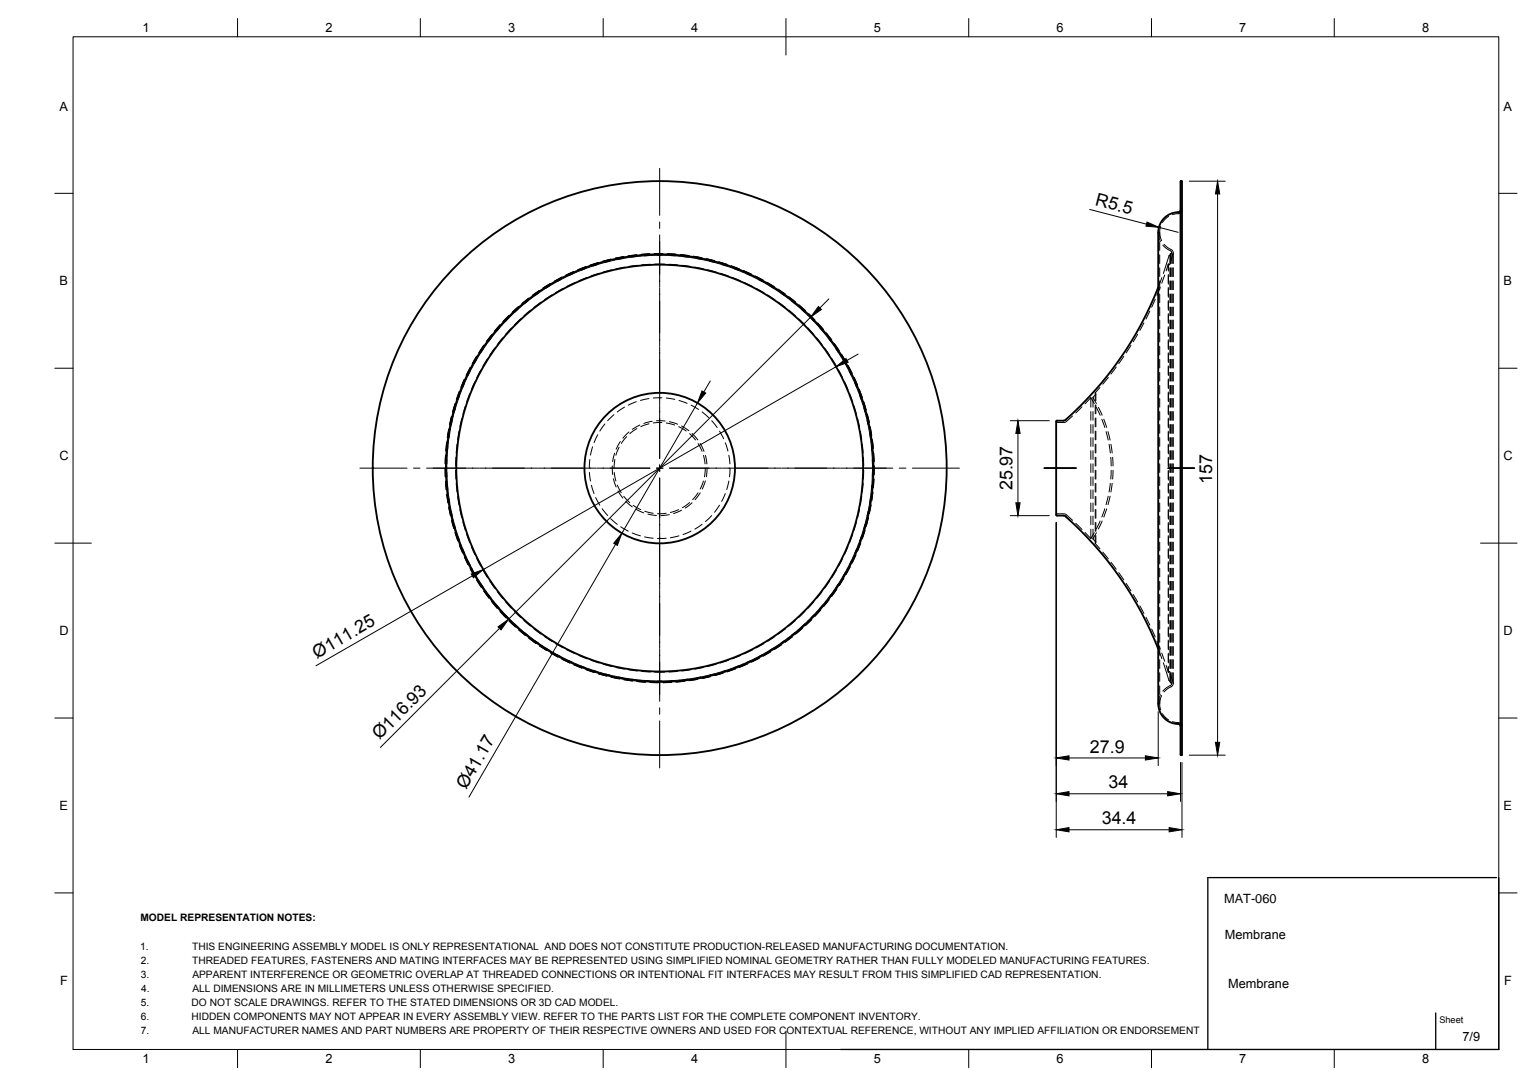
ISO-10303-21;
HEADER;
FILE_DESCRIPTION (('STEP AP214'),
    '1' );
FILE_NAME ('Membrane.step',
    '2026-10-29T23:46:56',
    ( '' ),
    ( '' ),
    'SwSTEP 2.0',
    'SolidWorks 2020',
    '' );
FILE_SCHEMA (( 'AUTOMOTIVE_DESIGN' ));
ENDSEC;

DATA;
#42=FILL_AREA_STYLE ('',( #30241 ) ) ;
#55=ORIENTED_EDGE ( 'NONE', *, *, #8639, .T. ) ;
#70=CIRCLE ( 'NONE', #12126, 59.80962967564905597 ) ;
#78=CARTESIAN_POINT ( 'NONE',  ( 21.09785597605719332, 15.24673779880127356, 47.04930799450051637 ) ) ;
#85=DIRECTION ( 'NONE',  ( 0.000000000000000000, 1.000000000000000000, -0.000000000000000000 ) ) ;
#87=AXIS2_PLACEMENT_3D ( 'NONE', #1243, #25723, #26032 ) ;
#88=DIRECTION ( 'NONE',  ( 0.000000000000000000, 1.000000000000000000, -0.000000000000000000 ) ) ;
#94=DIRECTION ( 'NONE',  ( 0.000000000000000000, 0.000000000000000000, 1.000000000000000000 ) ) ;
#128=DIRECTION ( 'NONE',  ( 0.000000000000000000, 0.000000000000000000, -1.000000000000000000 ) ) ;
#170=DIRECTION ( 'NONE',  ( -1.096245967261381435E-16, 0.000000000000000000, 1.000000000000000000 ) ) ;
#202=ORIENTED_EDGE ( 'NONE', *, *, #17749, .F. ) ;
#214=ORIENTED_EDGE ( 'NONE', *, *, #14166, .F. ) ;
#226=EDGE_CURVE ( 'NONE', #1958, #14944, #28442, .T. ) ;
#255=ORIENTED_EDGE ( 'NONE', *, *, #25304, .F. ) ;
#258=AXIS2_PLACEMENT_3D ( 'NONE', #29211, #16405, #11331 ) ;
#260=AXIS2_PLACEMENT_3D ( 'NONE', #19965, #12767, #2897 ) ;
#268=CARTESIAN_POINT ( 'NONE',  ( 21.09785597605719332, 14.58544108513610027, 34.31529089466609150 ) ) ;
#269=DIRECTION ( 'NONE',  ( -1.000000000000000000, 0.000000000000000000, 0.000000000000000000 ) ) ;
#307=CARTESIAN_POINT ( 'NONE',  ( 21.09785597605720042, -16.63545420775220407, -31.35069200549948221 ) ) ;
#329=EDGE_CURVE ( 'NONE', #6215, #18606, #11548, .T. ) ;
#347=DIRECTION ( 'NONE',  ( 0.000000000000000000, 0.000000000000000000, 1.000000000000000000 ) ) ;
#389=FACE_OUTER_BOUND ( 'NONE', #5612, .T. ) ;
#394=AXIS2_PLACEMENT_3D ( 'NONE', #24259, #4561, #23933 ) ;
#415=EDGE_LOOP ( 'NONE', ( #28557, #12550, #27414, #27034 ) ) ;
#427=DIRECTION ( 'NONE',  ( 0.000000000000000000, 0.000000000000000000, 1.000000000000000000 ) ) ;
#506=CARTESIAN_POINT ( 'NONE',  ( 21.09785597605719332, 14.77310068074637961, 33.81390520620020368 ) ) ;
#529=VERTEX_POINT ( 'NONE', #29166 ) ;
#549=ADVANCED_FACE ( 'NONE', ( #24556 ), #24396, .T. ) ;
#571=CARTESIAN_POINT ( 'NONE',  ( 21.09785597605719332, 7.237299147902269247, 47.04930799450051637 ) ) ;
#608=DIRECTION ( 'NONE',  ( 0.000000000000000000, 0.000000000000000000, -1.000000000000000000 ) ) ;
#653=CARTESIAN_POINT ( 'NONE',  ( 21.09785597605719332, 6.717634499306958773, 26.77287239547234066 ) ) ;
#660=AXIS2_PLACEMENT_3D ( 'NONE', #13969, #11830, #16569 ) ;
#664=CIRCLE ( 'NONE', #5918, 5.499019513592785735 ) ;
#673=CARTESIAN_POINT ( 'NONE',  ( -3.635677172050030048, -13.30632128221581212, 97.21573990761679340 ) ) ;
#675=DIRECTION ( 'NONE',  ( 0.000000000000000000, 0.000000000000000000, -1.000000000000000000 ) ) ;
#712=CIRCLE ( 'NONE', #19588, 0.6000000000000033085 ) ;
#722=CARTESIAN_POINT ( 'NONE',  ( 21.09785597605719332, 7.237299147902269247, 27.58963108451947832 ) ) ;
#726=DIRECTION ( 'NONE',  ( 0.000000000000000000, 0.000000000000000000, -1.000000000000000000 ) ) ;
#730=AXIS2_PLACEMENT_3D ( 'NONE', #24703, #6978, #12237 ) ;
#756=VERTEX_POINT ( 'NONE', #30915 ) ;
#769=CARTESIAN_POINT ( 'NONE',  ( 21.09785597605719332, 17.36451738380053555, 59.83349819502753775 ) ) ;
#806=DIRECTION ( 'NONE',  ( 0.000000000000000000, 0.000000000000000000, 1.000000000000000000 ) ) ;
#824=( GEOMETRIC_REPRESENTATION_CONTEXT ( 3 ) GLOBAL_UNCERTAINTY_ASSIGNED_CONTEXT ( ( #14065 ) ) GLOBAL_UNIT_ASSIGNED_CONTEXT ( ( #9888, #7594, #28105 ) ) REPRESENTATION_CONTEXT ( 'NONE', 'WORKASPACE' ) );
#834=DIRECTION ( 'NONE',  ( 0.000000000000000000, 0.000000000000000000, -1.000000000000000000 ) ) ;
#838=DIRECTION ( 'NONE',  ( 0.000000000000000000, 0.000000000000000000, -1.000000000000000000 ) ) ;
#846=CARTESIAN_POINT ( 'NONE',  ( 75.12562691325334185, -13.30632128221581212, 61.52060788219942822 ) ) ;
#851=CARTESIAN_POINT ( 'NONE',  ( 21.09785597605720042, -14.04221034894631615, -11.81388374861560386 ) ) ;
#989=CARTESIAN_POINT ( 'NONE',  ( -29.06857593705904108, -13.30632128221581212, 71.78284114260779347 ) ) ;
#994=CARTESIAN_POINT ( 'NONE',  ( 21.09785597605719332, 17.16451738380053271, 59.83349819502753775 ) ) ;
#1017=AXIS2_PLACEMENT_3D ( 'NONE', #653, #5424, #10682 ) ;
#1046=CARTESIAN_POINT ( 'NONE',  ( 21.09785597605720042, -16.73545420775220194, 47.04930799450051637 ) ) ;
#1047=DIRECTION ( 'NONE',  ( 0.000000000000000000, 0.000000000000000000, -1.000000000000000000 ) ) ;
#1059=DIRECTION ( 'NONE',  ( -0.000000000000000000, -1.000000000000000000, -0.000000000000000000 ) ) ;
#1070=EDGE_CURVE ( 'NONE', #20704, #4372, #13505, .T. ) ;
#1093=ORIENTED_EDGE ( 'NONE', *, *, #29693, .T. ) ;
#1113=DIRECTION ( 'NONE',  ( -0.000000000000000000, -1.000000000000000000, -0.000000000000000000 ) ) ;
#1117=EDGE_LOOP ( 'NONE', ( #3032, #2932, #25525, #9085 ) ) ;
#1139=AXIS2_PLACEMENT_3D ( 'NONE', #16369, #23761, #6373 ) ;
#1145=CARTESIAN_POINT ( 'NONE',  ( -27.33830150920369206, -13.30632128221581389, 19.07865907559173380 ) ) ;
#1157=VERTEX_POINT ( 'NONE', #4269 ) ;
#1163=EDGE_LOOP ( 'NONE', ( #13477, #4955, #25769, #255 ) ) ;
#1166=EDGE_CURVE ( 'NONE', #14445, #6352, #14609, .T. ) ;
#1168=FACE_OUTER_BOUND ( 'NONE', #32182, .T. ) ;
#1172=CARTESIAN_POINT ( 'NONE',  ( 21.09785597605720042, -14.54791319078308653, -11.41466734444011877 ) ) ;
#1181=AXIS2_PLACEMENT_3D ( 'NONE', #4062, #6693, #31807 ) ;
#1211=DIRECTION ( 'NONE',  ( 1.000000000000000000, 0.000000000000000000, 0.000000000000000000 ) ) ;
#1219=CARTESIAN_POINT ( 'NONE',  ( 21.09785597605719332, 17.16451738380053271, 47.04930799450051637 ) ) ;
#1243=CARTESIAN_POINT ( 'NONE',  ( 21.09785597605720753, -16.03545420775219910, 111.5493079945005235 ) ) ;
#1271=AXIS2_PLACEMENT_3D ( 'NONE', #17739, #12013, #20208 ) ;
#1318=ORIENTED_EDGE ( 'NONE', *, *, #9258, .F. ) ;
#1322=DIRECTION ( 'NONE',  ( -0.000000000000000000, -1.000000000000000000, -0.000000000000000000 ) ) ;
#1327=CARTESIAN_POINT ( 'NONE',  ( 39.85850837550805892, -13.74047052604243113, -8.200871005067009278 ) ) ;
#1354=DIRECTION ( 'NONE',  ( 0.000000000000000000, 0.000000000000000000, 1.000000000000000000 ) ) ;
#1374=DIRECTION ( 'NONE',  ( 0.000000000000000000, 0.000000000000000000, -1.000000000000000000 ) ) ;
#1376=ADVANCED_FACE ( 'NONE', ( #20171 ), #28437, .T. ) ;
#1399=EDGE_CURVE ( 'NONE', #18054, #15162, #3087, .T. ) ;
#1427=CARTESIAN_POINT ( 'NONE',  ( 21.09785597605720042, -13.37218737171702543, 47.04930799450051637 ) ) ;
#1455=DIRECTION ( 'NONE',  ( 0.000000000000000000, 1.000000000000000000, -0.000000000000000000 ) ) ;
#1456=CIRCLE ( 'NONE', #7745, 59.44168675549763492 ) ;
#1481=CARTESIAN_POINT ( 'NONE',  ( 76.91070899933976079, -13.30632128221581212, 43.39636530629569933 ) ) ;
#1486=CARTESIAN_POINT ( 'NONE',  ( 24.90860134598588616, -13.74047052604243468, -11.17459240441505841 ) ) ;
#1496=TOROIDAL_SURFACE ( 'NONE', #19845, 78.39999999999999147, 0.1000000000000014350 ) ;
#1506=AXIS2_PLACEMENT_3D ( 'NONE', #10006, #14769, #22786 ) ;
#1511=CARTESIAN_POINT ( 'NONE',  ( 21.09785597605720042, -17.03545420775220265, 47.04930799450051637 ) ) ;
#1520=DIRECTION ( 'NONE',  ( 3.629881133194233264E-17, 0.9550631830613039996, -0.2964022880492153122 ) ) ;
#1528=ORIENTED_EDGE ( 'NONE', *, *, #15802, .T. ) ;
#1531=DIRECTION ( 'NONE',  ( 1.000000000000000000, 0.000000000000000000, -1.224646799147353207E-16 ) ) ;
#1533=CARTESIAN_POINT ( 'NONE',  ( 21.09785597605720042, -13.68834655544033652, 47.04930799450051637 ) ) ;
#1540=AXIS2_PLACEMENT_3D ( 'NONE', #4446, #23662, #19040 ) ;
#1547=DIRECTION ( 'NONE',  ( 1.000000000000000000, 0.000000000000000000, -1.224646799147353207E-16 ) ) ;
#1549=CARTESIAN_POINT ( 'NONE',  ( 21.09785597605720753, -17.03545420775220265, 117.6483275080933169 ) ) ;
#1590=DIRECTION ( 'NONE',  ( -0.000000000000000000, -1.000000000000000000, -0.000000000000000000 ) ) ;
#1624=CIRCLE ( 'NONE', #32023, 69.59901951359279337 ) ;
#1655=CARTESIAN_POINT ( 'NONE',  ( 64.96297466771234497, -13.74047052604243646, 85.52521890125203186 ) ) ;
#1658=CARTESIAN_POINT ( 'NONE',  ( 21.09785597605720042, -13.64309448858209528, 47.04930799450051637 ) ) ;
#1672=FACE_OUTER_BOUND ( 'NONE', #25999, .T. ) ;
#1674=AXIS2_PLACEMENT_3D ( 'NONE', #9447, #19766, #14863 ) ;
#1683=ORIENTED_EDGE ( 'NONE', *, *, #28988, .F. ) ;
#1723=ORIENTED_EDGE ( 'NONE', *, *, #1399, .F. ) ;
#1735=AXIS2_PLACEMENT_3D ( 'NONE', #18661, #1113, #9306 ) ;
#1760=ORIENTED_EDGE ( 'NONE', *, *, #5361, .T. ) ;
#1806=ADVANCED_FACE ( 'NONE', ( #16019 ), #14235, .F. ) ;
#1807=CIRCLE ( 'NONE', #31687, 1.000000000000000888 ) ;
#1817=DIRECTION ( 'NONE',  ( 0.000000000000000000, 0.000000000000000000, -1.000000000000000000 ) ) ;
#1820=FACE_OUTER_BOUND ( 'NONE', #8386, .T. ) ;
#1832=FACE_OUTER_BOUND ( 'NONE', #19834, .T. ) ;
#1842=CARTESIAN_POINT ( 'NONE',  ( 21.09785597605719332, -13.74048473023143835, -11.17459240385188934 ) ) ;
#1846=ORIENTED_EDGE ( 'NONE', *, *, #12585, .F. ) ;
#1852=DIRECTION ( 'NONE',  ( 0.000000000000000000, 0.000000000000000000, -1.000000000000000000 ) ) ;
#1866=ORIENTED_EDGE ( 'NONE', *, *, #20239, .T. ) ;
#1904=AXIS2_PLACEMENT_3D ( 'NONE', #31595, #14029, #11568 ) ;
#1916=CARTESIAN_POINT ( 'NONE',  ( 1.883339950622007652, 7.264443105416139801, 47.04930799450051637 ) ) ;
#1942=CARTESIAN_POINT ( 'NONE',  ( 21.09785597605720042, -13.98292989133646103, 47.04930799450051637 ) ) ;
#1958=VERTEX_POINT ( 'NONE', #4188 ) ;
#1965=DIRECTION ( 'NONE',  ( 0.000000000000000000, 0.000000000000000000, -1.000000000000000000 ) ) ;
#1977=CARTESIAN_POINT ( 'NONE',  ( 39.85850837550807313, -13.74047052604243824, 102.2994869940680616 ) ) ;
#2054=DIRECTION ( 'NONE',  ( -0.000000000000000000, 0.000000000000000000, 1.000000000000000000 ) ) ;
#2060=DIRECTION ( 'NONE',  ( 0.000000000000000000, 1.000000000000000000, -0.000000000000000000 ) ) ;
#2074=AXIS2_PLACEMENT_3D ( 'NONE', #27150, #7137, #7301 ) ;
#2140=ORIENTED_EDGE ( 'NONE', *, *, #22896, .T. ) ;
#2158=AXIS2_PLACEMENT_3D ( 'NONE', #22995, #5122, #12845 ) ;
#2167=DIRECTION ( 'NONE',  ( 0.000000000000000000, 0.000000000000000000, 1.000000000000000000 ) ) ;
#2172=CARTESIAN_POINT ( 'NONE',  ( 21.09785597605719332, 6.547041198165487685, 47.04930799450051637 ) ) ;
#2203=DIRECTION ( 'NONE',  ( 1.169615070119505487E-16, -0.2964022880492245271, 0.9550631830613013351 ) ) ;
#2204=TOROIDAL_SURFACE ( 'NONE', #22655, 64.50000000000000000, 5.099019513592785380 ) ;
#2222=DIRECTION ( 'NONE',  ( 1.000000000000000000, 0.000000000000000000, -1.224646799147353207E-16 ) ) ;
#2226=DIRECTION ( 'NONE',  ( 0.000000000000000000, 0.000000000000000000, -1.000000000000000000 ) ) ;
#2233=PRODUCT_DEFINITION_SHAPE ( 'NONE', 'NONE',  #31780 ) ;
#2234=ORIENTED_EDGE ( 'NONE', *, *, #4882, .T. ) ;
#2241=ORIENTED_EDGE ( 'NONE', *, *, #24153, .T. ) ;
#2247=CIRCLE ( 'NONE', #18498, 55.68770647617149194 ) ;
#2292=ORIENTED_EDGE ( 'NONE', *, *, #24852, .F. ) ;
#2318=CARTESIAN_POINT ( 'NONE',  ( 21.09785597605719332, 17.36451738380053555, 47.04930799450051637 ) ) ;
#2320=CONICAL_SURFACE ( 'NONE', #20662, 58.70143199044622406, 1.269872874662816509 ) ;
#2330=CARTESIAN_POINT ( 'NONE',  ( 21.09785597605720042, -13.59284023713420630, 47.04930799450051637 ) ) ;
#2398=ORIENTED_EDGE ( 'NONE', *, *, #27659, .T. ) ;
#2399=CIRCLE ( 'NONE', #23356, 55.96105416618080142 ) ;
#2404=EDGE_CURVE ( 'NONE', #11885, #27524, #27429, .T. ) ;
#2428=DIRECTION ( 'NONE',  ( -1.000000000000000000, 0.000000000000000000, 0.000000000000000000 ) ) ;
#2447=CARTESIAN_POINT ( 'NONE',  ( 21.09785597605718976, 6.547041198165487685, 67.43013672359793986 ) ) ;
#2453=DIRECTION ( 'NONE',  ( -0.000000000000000000, -1.000000000000000000, -0.000000000000000000 ) ) ;
#2474=ORIENTED_EDGE ( 'NONE', *, *, #3629, .F. ) ;
#2484=EDGE_CURVE ( 'NONE', #20946, #18375, #23232, .T. ) ;
#2515=CIRCLE ( 'NONE', #13073, 58.84990142703892246 ) ;
#2542=CIRCLE ( 'NONE', #20877, 55.68770647617149194 ) ;
#2588=DIRECTION ( 'NONE',  ( 0.000000000000000000, 0.000000000000000000, -1.000000000000000000 ) ) ;
#2595=TOROIDAL_SURFACE ( 'NONE', #29318, 58.88977237527051756, 0.5999999999999987566 ) ;
#2596=ORIENTED_EDGE ( 'NONE', *, *, #6937, .F. ) ;
#2602=CIRCLE ( 'NONE', #5211, 19.45967690998103805 ) ;
#2607=ORIENTED_EDGE ( 'NONE', *, *, #8665, .T. ) ;
#2610=CARTESIAN_POINT ( 'NONE',  ( 21.09785597605720042, -13.87844638871996850, 47.04930799450051637 ) ) ;
#2628=CIRCLE ( 'NONE', #4190, 78.50000000000000000 ) ;
#2646=ORIENTED_EDGE ( 'NONE', *, *, #3109, .T. ) ;
#2653=CARTESIAN_POINT ( 'NONE',  ( 21.09785597605720753, -13.40182760052194588, 102.8325207889781439 ) ) ;
#2683=EDGE_CURVE ( 'NONE', #5958, #20704, #12223, .T. ) ;
#2745=DIRECTION ( 'NONE',  ( -0.000000000000000000, -1.000000000000000000, -0.000000000000000000 ) ) ;
#2768=VECTOR ( 'NONE', #3452, 1000.000000000000114 ) ;
#2774=DIRECTION ( 'NONE',  ( -1.169615070119510171E-16, -0.2964022880492104273, -0.9550631830613055540 ) ) ;
#2816=AXIS2_PLACEMENT_3D ( 'NONE', #19771, #27826, #2226 ) ;
#2853=AXIS2_PLACEMENT_3D ( 'NONE', #13835, #23830, #29087 ) ;
#2857=DIRECTION ( 'NONE',  ( 0.000000000000000000, -1.000000000000000000, 0.000000000000000000 ) ) ;
#2881=AXIS2_PLACEMENT_3D ( 'NONE', #2172, #32370, #4960 ) ;
#2884=AXIS2_PLACEMENT_3D ( 'NONE', #22880, #3008, #5170 ) ;
#2897=DIRECTION ( 'NONE',  ( 0.000000000000000000, 0.000000000000000000, -1.000000000000000000 ) ) ;
#2909=CIRCLE ( 'NONE', #25448, 94.44530576803552435 ) ;
#2918=VECTOR ( 'NONE', #6397, 1000.000000000000000 ) ;
#2932=ORIENTED_EDGE ( 'NONE', *, *, #9760, .T. ) ;
#2936=DIRECTION ( 'NONE',  ( 0.000000000000000000, 0.000000000000000000, -1.000000000000000000 ) ) ;
#2974=ORIENTED_EDGE ( 'NONE', *, *, #30326, .F. ) ;
#3008=DIRECTION ( 'NONE',  ( 0.000000000000000000, 1.000000000000000000, -0.000000000000000000 ) ) ;
#3009=ORIENTED_EDGE ( 'NONE', *, *, #27393, .F. ) ;
#3028=ORIENTED_EDGE ( 'NONE', *, *, #4339, .F. ) ;
#3029=CARTESIAN_POINT ( 'NONE',  ( 21.09785597605719687, -13.30631372918550959, -8.763520691563154941 ) ) ;
#3032=ORIENTED_EDGE ( 'NONE', *, *, #1070, .F. ) ;
#3042=AXIS2_PLACEMENT_3D ( 'NONE', #2653, #7742, #10050 ) ;
#3065=CIRCLE ( 'NONE', #25607, 78.39999999999999147 ) ;
#3067=CIRCLE ( 'NONE', #10926, 19.25826962553310295 ) ;
#3074=ORIENTED_EDGE ( 'NONE', *, *, #2484, .T. ) ;
#3075=DIRECTION ( 'NONE',  ( 0.000000000000000000, 1.000000000000000000, -0.000000000000000000 ) ) ;
#3077=AXIS2_PLACEMENT_3D ( 'NONE', #1533, #1059, #1374 ) ;
#3087=LINE ( 'NONE', #13127, #6941 ) ;
#3109=EDGE_CURVE ( 'NONE', #529, #11769, #28510, .T. ) ;
#3118=CARTESIAN_POINT ( 'NONE',  ( 21.09785597605720042, -13.59284023713420630, 47.04930799450051637 ) ) ;
#3147=TOROIDAL_SURFACE ( 'NONE', #7361, 19.31976987914897848, 0.2000000000000029809 ) ;
#3152=AXIS2_PLACEMENT_3D ( 'NONE', #1511, #6768, #28768 ) ;
#3196=CIRCLE ( 'NONE', #18902, 20.38082872909741994 ) ;
#3197=EDGE_LOOP ( 'NONE', ( #1318, #3565, #29612, #29507 ) ) ;
#3233=DIRECTION ( 'NONE',  ( 0.000000000000000000, 0.000000000000000000, -1.000000000000000000 ) ) ;
#3245=ORIENTED_EDGE ( 'NONE', *, *, #3999, .T. ) ;
#3288=CARTESIAN_POINT ( 'NONE',  ( -34.35522249183560461, -13.30632128221581389, 39.74351294429737891 ) ) ;
#3290=CARTESIAN_POINT ( 'NONE',  ( 99.49785597605720966, -17.03545420775220265, 47.04930799450051637 ) ) ;
#3293=CARTESIAN_POINT ( 'NONE',  ( 21.09785597605720042, -13.37218737171702543, 47.04930799450051637 ) ) ;
#3360=ORIENTED_EDGE ( 'NONE', *, *, #4615, .F. ) ;
#3365=FACE_OUTER_BOUND ( 'NONE', #21547, .T. ) ;
#3366=AXIS2_PLACEMENT_3D ( 'NONE', #9560, #6010, #28811 ) ;
#3385=CARTESIAN_POINT ( 'NONE',  ( 21.09785597605720042, -16.73545420775220194, 47.04930799450051637 ) ) ;
#3408=B_SPLINE_CURVE_WITH_KNOTS ( 'NONE', 3,
 ( #3626, #21171, #31209, #8717, #28427, #30573, #20864, #8087, #5941, #5779, #18397, #25790, #13338, #23335, #846, #10870, #4440, #1481, #21982, #3953, #14296, #16574, #26760, #11834, #9366, #16418, #13974, #14461, #23965, #9038, #4280, #31850, #11497, #26279 ),
 .UNSPECIFIED., .F., .F.,
 ( 4, 2, 2, 2, 2, 2, 2, 2, 2, 2, 2, 2, 2, 2, 2, 2, 4 ),
 ( 0.5000000000000000000, 0.5312500000000000000, 0.5625000000000000000, 0.5937500000000000000, 0.6250000000000000000, 0.6562500000000000000, 0.6875000000000001110, 0.7187500000000002220, 0.7500000000000002220, 0.7812500000000002220, 0.8125000000000002220, 0.8437500000000002220, 0.8750000000000002220, 0.9062500000000002220, 0.9375000000000001110, 0.9687500000000000000, 1.000000000000000000 ),
 .UNSPECIFIED. ) ;
#3414=CIRCLE ( 'NONE', #18103, 58.46397533894063514 ) ;
#3420=CIRCLE ( 'NONE', #23346, 20.58349629884742882 ) ;
#3421=ORIENTED_EDGE ( 'NONE', *, *, #5597, .T. ) ;
#3450=CARTESIAN_POINT ( 'NONE',  ( -15.78477032795855273, -13.30632128221581034, 5.000640598253890623 ) ) ;
#3452=DIRECTION ( 'NONE',  ( 0.000000000000000000, 0.9550631830612811290, 0.2964022880492887535 ) ) ;
#3453=ORIENTED_EDGE ( 'NONE', *, *, #12042, .F. ) ;
#3454=DIRECTION ( 'NONE',  ( 0.000000000000000000, 0.000000000000000000, 1.000000000000000000 ) ) ;
#3455=ORIENTED_EDGE ( 'NONE', *, *, #20389, .T. ) ;
#3457=FACE_OUTER_BOUND ( 'NONE', #20170, .T. ) ;
#3501=ORIENTED_EDGE ( 'NONE', *, *, #25610, .F. ) ;
#3531=DIRECTION ( 'NONE',  ( 0.000000000000000000, 1.000000000000000000, -0.000000000000000000 ) ) ;
#3536=FACE_OUTER_BOUND ( 'NONE', #12646, .T. ) ;
#3540=ORIENTED_EDGE ( 'NONE', *, *, #15853, .F. ) ;
#3544=CARTESIAN_POINT ( 'NONE',  ( 21.09785597605717555, 77.37241625295546044, 131.0041668858331150 ) ) ;
#3565=ORIENTED_EDGE ( 'NONE', *, *, #9477, .F. ) ;
#3573=EDGE_LOOP ( 'NONE', ( #10658, #5418, #25603, #19859 ) ) ;
#3602=AXIS2_PLACEMENT_3D ( 'NONE', #4162, #14189, #1211 ) ;
#3603=CIRCLE ( 'NONE', #20350, 58.09216821878681003 ) ;
#3611=CARTESIAN_POINT ( 'NONE',  ( -12.94741462430177315, -13.30632128221581389, 2.672082950226038367 ) ) ;
#3626=CARTESIAN_POINT ( 'NONE',  ( 21.09785597605719687, -13.30631372918550959, 102.8621366805641770 ) ) ;
#3629=EDGE_CURVE ( 'NONE', #27949, #20704, #24670, .T. ) ;
#3645=LINE ( 'NONE', #25811, #24845 ) ;
#3675=CIRCLE ( 'NONE', #3152, 70.59901951359279337 ) ;
#3686=AXIS2_PLACEMENT_3D ( 'NONE', #10722, #30256, #30584 ) ;
#3703=DIRECTION ( 'NONE',  ( 0.000000000000000000, 0.000000000000000000, -1.000000000000000000 ) ) ;
#3735=DIRECTION ( 'NONE',  ( 0.000000000000000000, 0.000000000000000000, -1.000000000000000000 ) ) ;
#3760=AXIS2_PLACEMENT_3D ( 'NONE', #7446, #17441, #24497 ) ;
#3772=CARTESIAN_POINT ( 'NONE',  ( -12.94741462430176249, -13.30632128221581212, 91.42653303877501969 ) ) ;
#3773=CIRCLE ( 'NONE', #3760, 78.39999999999999147 ) ;
#3784=ORIENTED_EDGE ( 'NONE', *, *, #31237, .F. ) ;
#3785=ORIENTED_EDGE ( 'NONE', *, *, #9760, .F. ) ;
#3792=CARTESIAN_POINT ( 'NONE',  ( 28.71925248772579664, -13.74047052604243291, -10.79927602576051093 ) ) ;
#3800=ADVANCED_FACE ( 'NONE', ( #1820 ), #8372, .F. ) ;
#3802=CARTESIAN_POINT ( 'NONE',  ( 21.09785597605719332, 38.31023907818019580, 47.04930799450051637 ) ) ;
#3813=CARTESIAN_POINT ( 'NONE',  ( 21.09785597605721108, -16.73545420775220194, 125.5493079945005093 ) ) ;
#3822=EDGE_CURVE ( 'NONE', #18054, #23177, #20677, .T. ) ;
#3843=CIRCLE ( 'NONE', #1735, 55.62393233686778160 ) ;
#3864=VERTEX_POINT ( 'NONE', #22325 ) ;
#3915=CIRCLE ( 'NONE', #26990, 78.50000000000000000 ) ;
#3918=AXIS2_PLACEMENT_3D ( 'NONE', #26048, #3075, #30672 ) ;
#3942=ORIENTED_EDGE ( 'NONE', *, *, #14008, .F. ) ;
#3943=CARTESIAN_POINT ( 'NONE',  ( -34.71499704722533153, -13.30632128221581034, 50.70225068270534052 ) ) ;
#3953=CARTESIAN_POINT ( 'NONE',  ( 75.12562691325332764, -13.30632128221581212, 32.57800810680159032 ) ) ;
#3959=CARTESIAN_POINT ( 'NONE',  ( 67.39212317433589305, -13.74047052604243824, 11.53332310724655230 ) ) ;
#3974=ORIENTED_EDGE ( 'NONE', *, *, #10954, .T. ) ;
#3989=DIRECTION ( 'NONE',  ( 0.000000000000000000, 0.000000000000000000, -1.000000000000000000 ) ) ;
#3999=EDGE_CURVE ( 'NONE', #9462, #25082, #8400, .T. ) ;
#4050=DIRECTION ( 'NONE',  ( 0.000000000000000000, 1.000000000000000000, -0.000000000000000000 ) ) ;
#4054=EDGE_LOOP ( 'NONE', ( #31986, #7662, #22931, #16979 ) ) ;
#4062=CARTESIAN_POINT ( 'NONE',  ( 99.49785597605720966, -16.63545420775220052, 47.04930799450051637 ) ) ;
#4113=CARTESIAN_POINT ( 'NONE',  ( 59.57376688280871946, -13.74047052604243646, 3.184189302845370495 ) ) ;
#4116=DIRECTION ( 'NONE',  ( 0.000000000000000000, 1.000000000000000000, -0.000000000000000000 ) ) ;
#4121=CARTESIAN_POINT ( 'NONE',  ( 21.09785597605720753, -13.59284023713420630, 102.7732403313682994 ) ) ;
#4135=AXIS2_PLACEMENT_3D ( 'NONE', #7384, #2453, #12470 ) ;
#4141=DIRECTION ( 'NONE',  ( 0.000000000000000000, 0.000000000000000000, -1.000000000000000000 ) ) ;
#4162=CARTESIAN_POINT ( 'NONE',  ( 21.09785597605719332, 38.31023907818019580, 47.04930799450051637 ) ) ;
#4188=CARTESIAN_POINT ( 'NONE',  ( 21.09785597605721108, -16.63545420775220407, 125.4493079945005150 ) ) ;
#4190=AXIS2_PLACEMENT_3D ( 'NONE', #30921, #5814, #25981 ) ;
#4223=AXIS2_PLACEMENT_3D ( 'NONE', #9362, #19356, #15573 ) ;
#4259=CARTESIAN_POINT ( 'NONE',  ( 21.09785597605719332, 34.11266481626051217, 47.04930799450051637 ) ) ;
#4264=ADVANCED_FACE ( 'NONE', ( #30492 ), #22563, .F. ) ;
#4269=CARTESIAN_POINT ( 'NONE',  ( 21.09785597605719332, 6.671061906060458568, 26.46581169565308755 ) ) ;
#4278=ORIENTED_EDGE ( 'NONE', *, *, #10988, .F. ) ;
#4280=CARTESIAN_POINT ( 'NONE',  ( 35.56915586375611582, -13.30632128221581212, -6.978462942695603743 ) ) ;
#4302=DIRECTION ( 'NONE',  ( 0.000000000000000000, 0.000000000000000000, -1.000000000000000000 ) ) ;
#4303=CARTESIAN_POINT ( 'NONE',  ( 21.09785597605720042, -13.37218737171702543, 47.04930799450051637 ) ) ;
#4331=ORIENTED_EDGE ( 'NONE', *, *, #31682, .T. ) ;
#4339=EDGE_CURVE ( 'NONE', #29876, #31613, #29914, .T. ) ;
#4351=CARTESIAN_POINT ( 'NONE',  ( 21.09785597605720042, -16.03545420775219910, 47.04930799450051637 ) ) ;
#4372=VERTEX_POINT ( 'NONE', #769 ) ;
#4389=DIRECTION ( 'NONE',  ( 0.000000000000000000, 0.000000000000000000, 1.000000000000000000 ) ) ;
#4407=CIRCLE ( 'NONE', #18609, 78.39999999999999147 ) ;
#4431=CARTESIAN_POINT ( 'NONE',  ( 21.09785597605719332, -13.49020584019834601, 105.1414762132873193 ) ) ;
#4435=FACE_OUTER_BOUND ( 'NONE', #24062, .T. ) ;
#4440=CARTESIAN_POINT ( 'NONE',  ( 76.91070899933976079, -13.30632128221581212, 50.70225068270534763 ) ) ;
#4446=CARTESIAN_POINT ( 'NONE',  ( 21.09785597605720042, -13.37218737171702543, 47.04930799450051637 ) ) ;
#4467=CARTESIAN_POINT ( 'NONE',  ( 21.09785597605719332, 17.16451738380053271, 47.04930799450051637 ) ) ;
#4485=CARTESIAN_POINT ( 'NONE',  ( 21.09785597605719332, 14.58544108513610027, 59.78332509433494124 ) ) ;
#4534=AXIS2_PLACEMENT_3D ( 'NONE', #19092, #14200, #29129 ) ;
#4545=EDGE_CURVE ( 'NONE', #14867, #11885, #26250, .T. ) ;
#4560=DIRECTION ( 'NONE',  ( 0.000000000000000000, 0.000000000000000000, -1.000000000000000000 ) ) ;
#4561=DIRECTION ( 'NONE',  ( 0.000000000000000000, -1.000000000000000000, 0.000000000000000000 ) ) ;
#4570=ORIENTED_EDGE ( 'NONE', *, *, #2683, .T. ) ;
#4582=EDGE_LOOP ( 'NONE', ( #10714, #25149, #27986, #22308 ) ) ;
#4607=ADVANCED_FACE ( 'NONE', ( #32423 ), #32015, .F. ) ;
#4615=EDGE_CURVE ( 'NONE', #28177, #11145, #22044, .T. ) ;
#4645=CARTESIAN_POINT ( 'NONE',  ( 21.09785597605719332, 17.16451738380053271, 34.26511779397349500 ) ) ;
#4652=DIRECTION ( 'NONE',  ( 0.000000000000000000, 0.000000000000000000, -1.000000000000000000 ) ) ;
#4657=ORIENTED_EDGE ( 'NONE', *, *, #31935, .F. ) ;
#4668=ORIENTED_EDGE ( 'NONE', *, *, #7760, .T. ) ;
#4681=DIRECTION ( 'NONE',  ( 0.000000000000000000, 0.000000000000000000, -1.000000000000000000 ) ) ;
#4683=FACE_OUTER_BOUND ( 'NONE', #31207, .T. ) ;
#4690=CIRCLE ( 'NONE', #10465, 0.1999999999999987899 ) ;
#4698=CONICAL_SURFACE ( 'NONE', #16239, 20.38082872909741994, 1.021642509542357802 ) ;
#4712=ORIENTED_EDGE ( 'NONE', *, *, #3629, .T. ) ;
#4727=DIRECTION ( 'NONE',  ( 0.000000000000000000, 1.000000000000000000, -0.000000000000000000 ) ) ;
#4760=TOROIDAL_SURFACE ( 'NONE', #10014, 58.86319174311611846, 0.1999999999999984290 ) ;
#4781=DIRECTION ( 'NONE',  ( -1.000000000000000000, 0.000000000000000000, 0.000000000000000000 ) ) ;
#4797=CARTESIAN_POINT ( 'NONE',  ( -25.19641122222149576, -13.74047052604243646, 82.56529288175448755 ) ) ;
#4852=CARTESIAN_POINT ( 'NONE',  ( 21.09785597605719332, 6.717634499306958773, 47.04930799450051637 ) ) ;
#4857=ADVANCED_FACE ( 'NONE', ( #16457 ), #19772, .T. ) ;
#4858=CARTESIAN_POINT ( 'NONE',  ( 21.09785597605720042, -16.03545420775219910, -17.45069200549948718 ) ) ;
#4865=EDGE_LOOP ( 'NONE', ( #26649, #31897, #11347, #7235 ) ) ;
#4873=CIRCLE ( 'NONE', #31611, 0.1000000000000011297 ) ;
#4875=CARTESIAN_POINT ( 'NONE',  ( 21.09785597605719332, 38.31023907818019580, 47.04930799450051637 ) ) ;
#4882=EDGE_CURVE ( 'NONE', #31146, #14944, #16628, .T. ) ;
#4899=DIRECTION ( 'NONE',  ( -0.000000000000000000, -1.000000000000000000, -0.000000000000000000 ) ) ;
#4905=EDGE_CURVE ( 'NONE', #20809, #32483, #26149, .T. ) ;
#4906=CIRCLE ( 'NONE', #32155, 20.38082872909741994 ) ;
#4911=EDGE_LOOP ( 'NONE', ( #8926, #30976, #16052, #8516 ) ) ;
#4940=DIRECTION ( 'NONE',  ( 0.000000000000000000, 0.000000000000000000, -1.000000000000000000 ) ) ;
#4955=ORIENTED_EDGE ( 'NONE', *, *, #15318, .T. ) ;
#4960=DIRECTION ( 'NONE',  ( 0.000000000000000000, 0.000000000000000000, -1.000000000000000000 ) ) ;
#4975=AXIS2_PLACEMENT_3D ( 'NONE', #27104, #17418, #14969 ) ;
#4984=AXIS2_PLACEMENT_3D ( 'NONE', #3293, #15775, #347 ) ;
#4988=AXIS2_PLACEMENT_3D ( 'NONE', #11967, #13956, #23947 ) ;
#4999=CIRCLE ( 'NONE', #25373, 20.58349629884742882 ) ;
#5020=CARTESIAN_POINT ( 'NONE',  ( 21.09785597605720042, -13.68834655544033652, 47.04930799450051637 ) ) ;
#5031=COLOUR_RGB ( '',0.7921568627450980005, 0.8196078431372548767, 0.9333333333333333481 ) ;
#5037=EDGE_CURVE ( 'NONE', #29666, #18375, #30289, .T. ) ;
#5062=CYLINDRICAL_SURFACE ( 'NONE', #6403, 78.50000000000000000 ) ;
#5085=DIRECTION ( 'NONE',  ( 0.000000000000000000, 1.000000000000000000, -0.000000000000000000 ) ) ;
#5094=CARTESIAN_POINT ( 'NONE',  ( 21.09785597605720042, -14.24176827912842391, 47.04930799450051637 ) ) ;
#5103=ORIENTED_EDGE ( 'NONE', *, *, #2404, .T. ) ;
#5107=CIRCLE ( 'NONE', #15592, 0.1999999999999987899 ) ;
#5118=AXIS2_PLACEMENT_3D ( 'NONE', #5677, #23715, #18461 ) ;
#5122=DIRECTION ( 'NONE',  ( 0.000000000000000000, 1.000000000000000000, -0.000000000000000000 ) ) ;
#5137=DIRECTION ( 'NONE',  ( 0.000000000000000000, 0.000000000000000000, -1.000000000000000000 ) ) ;
#5144=CARTESIAN_POINT ( 'NONE',  ( 21.09785597605720042, -16.03545420775220265, -22.54971151909227700 ) ) ;
#5170=DIRECTION ( 'NONE',  ( 0.000000000000000000, 0.000000000000000000, -1.000000000000000000 ) ) ;
#5211=AXIS2_PLACEMENT_3D ( 'NONE', #571, #13061, #10763 ) ;
#5212=DIRECTION ( 'NONE',  ( -0.000000000000000000, -1.000000000000000000, -0.000000000000000000 ) ) ;
#5222=DIRECTION ( 'NONE',  ( 0.000000000000000000, 0.000000000000000000, -1.000000000000000000 ) ) ;
#5248=EDGE_LOOP ( 'NONE', ( #4570, #8141, #13699, #32453 ) ) ;
#5278=CARTESIAN_POINT ( 'NONE',  ( 21.09785597605718976, 7.264443105416139801, 66.26382401993569715 ) ) ;
#5292=FACE_OUTER_BOUND ( 'NONE', #4582, .T. ) ;
#5297=ORIENTED_EDGE ( 'NONE', *, *, #22376, .F. ) ;
#5322=CONICAL_SURFACE ( 'NONE', #12136, 58.70143199044622406, 1.269872874662816509 ) ;
#5335=DIRECTION ( 'NONE',  ( 0.000000000000000000, 0.000000000000000000, -1.000000000000000000 ) ) ;
#5361=EDGE_CURVE ( 'NONE', #29666, #27949, #9849, .T. ) ;
#5376=DIRECTION ( 'NONE',  ( -0.000000000000000000, -1.000000000000000000, -0.000000000000000000 ) ) ;
#5395=ORIENTED_EDGE ( 'NONE', *, *, #21571, .F. ) ;
#5409=ORIENTED_EDGE ( 'NONE', *, *, #30326, .T. ) ;
#5418=ORIENTED_EDGE ( 'NONE', *, *, #22376, .T. ) ;
#5424=DIRECTION ( 'NONE',  ( 1.000000000000000000, 0.000000000000000000, 0.000000000000000000 ) ) ;
#5449=DIRECTION ( 'NONE',  ( 0.000000000000000000, 0.000000000000000000, -1.000000000000000000 ) ) ;
#5463=EDGE_CURVE ( 'NONE', #17607, #29601, #8013, .T. ) ;
#5477=ORIENTED_EDGE ( 'NONE', *, *, #22080, .F. ) ;
#5485=DIRECTION ( 'NONE',  ( 0.000000000000000000, 0.000000000000000000, -1.000000000000000000 ) ) ;
#5486=CIRCLE ( 'NONE', #4975, 1.000000000001013856 ) ;
#5491=ORIENTED_EDGE ( 'NONE', *, *, #26667, .T. ) ;
#5520=DIRECTION ( 'NONE',  ( 3.629881133195132442E-17, 0.9550631830612811290, -0.2964022880492887535 ) ) ;
#5521=ORIENTED_EDGE ( 'NONE', *, *, #329, .T. ) ;
#5560=ADVANCED_FACE ( 'NONE', ( #22769 ), #27175, .T. ) ;
#5577=EDGE_CURVE ( 'NONE', #11769, #22362, #3067, .T. ) ;
#5597=EDGE_CURVE ( 'NONE', #29666, #5958, #15880, .T. ) ;
#5612=EDGE_LOOP ( 'NONE', ( #12655, #6042 ) ) ;
#5649=AXIS2_PLACEMENT_3D ( 'NONE', #8838, #8361, #18358 ) ;
#5677=CARTESIAN_POINT ( 'NONE',  ( 21.09785597605719332, 38.31023907818019580, 47.04930799450051637 ) ) ;
#5691=CARTESIAN_POINT ( 'NONE',  ( 21.09785597605720042, -16.03545420775220265, 47.04930799450051637 ) ) ;
#5701=CARTESIAN_POINT ( 'NONE',  ( 21.09785597605719332, 7.881678200673685630, 47.04930799450051637 ) ) ;
#5757=ORIENTED_EDGE ( 'NONE', *, *, #12585, .T. ) ;
#5771=CARTESIAN_POINT ( 'NONE',  ( 21.09785597605719332, -13.49020584019834601, -11.04286022428629188 ) ) ;
#5779=CARTESIAN_POINT ( 'NONE',  ( 63.14652337230385371, -13.30632128221581389, 83.93193429851626775 ) ) ;
#5814=DIRECTION ( 'NONE',  ( -0.000000000000000000, -1.000000000000000000, -0.000000000000000000 ) ) ;
#5832=DIRECTION ( 'NONE',  ( -1.000000000000000000, 0.000000000000000000, -1.224646799147353207E-16 ) ) ;
#5834=ADVANCED_FACE ( 'NONE', ( #32271 ), #19941, .F. ) ;
#5835=CARTESIAN_POINT ( 'NONE',  ( 21.09785597605720042, -13.64309448858209528, -11.84046438077000118 ) ) ;
#5840=AXIS2_PLACEMENT_3D ( 'NONE', #23735, #8648, #13421 ) ;
#5846=EDGE_CURVE ( 'NONE', #30037, #14004, #22456, .T. ) ;
#5851=CARTESIAN_POINT ( 'NONE',  ( 21.09785597605720042, -13.59284023713420630, 47.04930799450051637 ) ) ;
#5888=ORIENTED_EDGE ( 'NONE', *, *, #15318, .F. ) ;
#5896=DIRECTION ( 'NONE',  ( 0.000000000000000000, -0.2964022880492265255, -0.9550631830613005580 ) ) ;
#5904=DIRECTION ( 'NONE',  ( -1.000000000000000000, 0.000000000000000000, -1.224646799147353207E-16 ) ) ;
#5908=EDGE_CURVE ( 'NONE', #29601, #20020, #14648, .T. ) ;
#5918=AXIS2_PLACEMENT_3D ( 'NONE', #4858, #25204, #94 ) ;
#5941=CARTESIAN_POINT ( 'NONE',  ( 57.98048228007294114, -13.30632128221581212, 89.09797539074718031 ) ) ;
#5943=EDGE_CURVE ( 'NONE', #24037, #17607, #2602, .T. ) ;
#5958=VERTEX_POINT ( 'NONE', #30137 ) ;
#5977=DIRECTION ( 'NONE',  ( 1.000000000000000000, 0.000000000000000000, 0.000000000000000000 ) ) ;
#5978=ORIENTED_EDGE ( 'NONE', *, *, #32402, .F. ) ;
#5986=EDGE_LOOP ( 'NONE', ( #20602, #9686, #13312, #23710 ) ) ;
#5991=ORIENTED_EDGE ( 'NONE', *, *, #20389, .F. ) ;
#6000=AXIS2_PLACEMENT_3D ( 'NONE', #4875, #427, #269 ) ;
#6004=EDGE_CURVE ( 'NONE', #14867, #27708, #4690, .T. ) ;
#6010=DIRECTION ( 'NONE',  ( -0.000000000000000000, -1.000000000000000000, -0.000000000000000000 ) ) ;
#6028=EDGE_CURVE ( 'NONE', #29052, #14004, #29860, .T. ) ;
#6029=DIRECTION ( 'NONE',  ( 0.000000000000000000, -0.6995351541602693457, 0.7145981864614324719 ) ) ;
#6042=ORIENTED_EDGE ( 'NONE', *, *, #14998, .T. ) ;
#6074=AXIS2_PLACEMENT_3D ( 'NONE', #15977, #28615, #726 ) ;
#6145=EDGE_LOOP ( 'NONE', ( #24417, #30662, #26066, #7969 ) ) ;
#6186=VECTOR ( 'NONE', #5520, 1000.000000000000114 ) ;
#6191=ORIENTED_EDGE ( 'NONE', *, *, #26529, .T. ) ;
#6213=DIRECTION ( 'NONE',  ( 0.000000000000000000, 0.000000000000000000, 1.000000000000000000 ) ) ;
#6215=VERTEX_POINT ( 'NONE', #24675 ) ;
#6223=ORIENTED_EDGE ( 'NONE', *, *, #5463, .T. ) ;
#6225=VERTEX_POINT ( 'NONE', #14999 ) ;
#6257=EDGE_CURVE ( 'NONE', #1157, #6923, #31951, .T. ) ;
#6261=ORIENTED_EDGE ( 'NONE', *, *, #10555, .F. ) ;
#6262=DIRECTION ( 'NONE',  ( 0.000000000000000000, 1.000000000000000000, -0.000000000000000000 ) ) ;
#6279=VECTOR ( 'NONE', #22851, 1000.000000000000000 ) ;
#6286=CARTESIAN_POINT ( 'NONE',  ( 0.000000000000000000, 0.000000000000000000, 0.000000000000000000 ) ) ;
#6297=CARTESIAN_POINT ( 'NONE',  ( 21.09785597605720753, -16.03545420775220265, 116.6483275080933169 ) ) ;
#6302=CIRCLE ( 'NONE', #27794, 20.13652856819611969 ) ;
#6307=ORIENTED_EDGE ( 'NONE', *, *, #15631, .F. ) ;
#6320=FACE_OUTER_BOUND ( 'NONE', #26532, .T. ) ;
#6331=FACE_OUTER_BOUND ( 'NONE', #21498, .T. ) ;
#6332=AXIS2_PLACEMENT_3D ( 'NONE', #15383, #28182, #15869 ) ;
#6352=VERTEX_POINT ( 'NONE', #19699 ) ;
#6363=CARTESIAN_POINT ( 'NONE',  ( 21.09785597605719332, 17.16451738380053627, 47.04930799450051637 ) ) ;
#6373=DIRECTION ( 'NONE',  ( 0.000000000000000000, 0.000000000000000000, -1.000000000000000000 ) ) ;
#6378=CARTESIAN_POINT ( 'NONE',  ( 21.09785597605719332, 17.16451738380053627, 59.73344952167762756 ) ) ;
#6397=DIRECTION ( 'NONE',  ( 0.000000000000000000, 0.5219656503457801300, -0.8529665057076430967 ) ) ;
#6402=CARTESIAN_POINT ( 'NONE',  ( 21.09785597605719332, 7.094379510609982731, 27.72953811535153079 ) ) ;
#6403=AXIS2_PLACEMENT_3D ( 'NONE', #9822, #15073, #19819 ) ;
#6450=CARTESIAN_POINT ( 'NONE',  ( 21.09785597605719332, 6.574714862014670480, 47.04930799450051637 ) ) ;
#6453=DIRECTION ( 'NONE',  ( -0.000000000000000000, -1.000000000000000000, -0.000000000000000000 ) ) ;
#6481=EDGE_CURVE ( 'NONE', #15416, #14823, #17204, .T. ) ;
#6503=FACE_OUTER_BOUND ( 'NONE', #25846, .T. ) ;
#6523=EDGE_CURVE ( 'NONE', #6567, #24849, #20889, .T. ) ;
#6525=CARTESIAN_POINT ( 'NONE',  ( 21.09785597605720042, -13.64309448858209528, 47.04930799450051637 ) ) ;
#6535=DIRECTION ( 'NONE',  ( 1.000000000000000000, 0.000000000000000000, 0.000000000000000000 ) ) ;
#6539=DIRECTION ( 'NONE',  ( 0.000000000000000000, 1.000000000000000000, -0.000000000000000000 ) ) ;
#6543=CARTESIAN_POINT ( 'NONE',  ( 21.09785597605718621, 6.547041198165487685, 67.43013672359793986 ) ) ;
#6567=VERTEX_POINT ( 'NONE', #26248 ) ;
#6576=CARTESIAN_POINT ( 'NONE',  ( 21.09785597605719332, 38.31023907818019580, 47.04930799450051637 ) ) ;
#6587=CARTESIAN_POINT ( 'NONE',  ( 79.32175637497277876, -13.74047052604243646, 50.86005336442920566 ) ) ;
#6610=CARTESIAN_POINT ( 'NONE',  ( -25.19641122222150287, -13.74047052604243646, 11.53332310724657539 ) ) ;
#6627=FACE_OUTER_BOUND ( 'NONE', #28071, .T. ) ;
#6637=EDGE_LOOP ( 'NONE', ( #14247, #23679 ) ) ;
#6640=LINE ( 'NONE', #6797, #17899 ) ;
#6677=AXIS2_PLACEMENT_3D ( 'NONE', #31573, #15826, #3989 ) ;
#6693=DIRECTION ( 'NONE',  ( 0.000000000000000000, 1.000000000000000000, 0.000000000000000000 ) ) ;
#6702=AXIS2_PLACEMENT_3D ( 'NONE', #30306, #7328, #9954 ) ;
#6727=DIRECTION ( 'NONE',  ( 0.000000000000000000, -0.2964022880492104273, 0.9550631830613055540 ) ) ;
#6730=DIRECTION ( 'NONE',  ( -1.000000000000000000, 0.000000000000000000, 0.000000000000000000 ) ) ;
#6736=ADVANCED_FACE ( 'NONE', ( #7491 ), #30347, .T. ) ;
#6742=CARTESIAN_POINT ( 'NONE',  ( 78.94643999631823306, -13.74047052604243646, 54.67070450616910904 ) ) ;
#6743=ORIENTED_EDGE ( 'NONE', *, *, #5577, .T. ) ;
#6761=CARTESIAN_POINT ( 'NONE',  ( 21.09785597605720753, -13.88867167006704939, -11.65212399594570769 ) ) ;
#6767=CARTESIAN_POINT ( 'NONE',  ( -35.26384896152210757, -13.74047052604243646, 62.14575043855078462 ) ) ;
#6768=DIRECTION ( 'NONE',  ( -0.000000000000000000, -1.000000000000000000, -0.000000000000000000 ) ) ;
#6774=EDGE_CURVE ( 'NONE', #27708, #27524, #24057, .T. ) ;
#6792=ORIENTED_EDGE ( 'NONE', *, *, #24153, .F. ) ;
#6797=CARTESIAN_POINT ( 'NONE',  ( 21.09785597605720753, -13.68834655544033652, 102.7436001025633772 ) ) ;
#6808=DIRECTION ( 'NONE',  ( 0.000000000000000000, 0.000000000000000000, -1.000000000000000000 ) ) ;
#6811=DIRECTION ( 'NONE',  ( -0.000000000000000000, -1.000000000000000000, -0.000000000000000000 ) ) ;
#6858=( GEOMETRIC_REPRESENTATION_CONTEXT ( 3 ) GLOBAL_UNCERTAINTY_ASSIGNED_CONTEXT ( ( #19289 ) ) GLOBAL_UNIT_ASSIGNED_CONTEXT ( ( #28350, #15874, #19449 ) ) REPRESENTATION_CONTEXT ( 'NONE', 'WORKASPACE' ) );
#6869=ORIENTED_EDGE ( 'NONE', *, *, #3822, .T. ) ;
#6892=DIRECTION ( 'NONE',  ( 0.000000000000000000, 0.000000000000000000, 1.000000000000000000 ) ) ;
#6913=AXIS2_PLACEMENT_3D ( 'NONE', #29836, #12605, #29512 ) ;
#6923=VERTEX_POINT ( 'NONE', #3029 ) ;
#6931=CARTESIAN_POINT ( 'NONE',  ( -22.76726271559793702, -13.74047052604243646, 85.52521890125204607 ) ) ;
#6937=EDGE_CURVE ( 'NONE', #14823, #15416, #17760, .T. ) ;
#6941=VECTOR ( 'NONE', #5896, 1000.000000000000341 ) ;
#6974=ADVANCED_FACE ( 'NONE', ( #26329 ), #19339, .T. ) ;
#6976=ORIENTED_EDGE ( 'NONE', *, *, #28609, .F. ) ;
#6978=DIRECTION ( 'NONE',  ( 1.000000000000000000, 0.000000000000000000, -1.224646799147353207E-16 ) ) ;
#6981=DIRECTION ( 'NONE',  ( 0.000000000000000000, 1.000000000000000000, -0.000000000000000000 ) ) ;
#6983=AXIS2_PLACEMENT_3D ( 'NONE', #23128, #18671, #28693 ) ;
#6986=LINE ( 'NONE', #31773, #18413 ) ;
#6996=ADVANCED_FACE ( 'NONE', ( #13705 ), #28961, .F. ) ;
#7007=AXIS2_PLACEMENT_3D ( 'NONE', #29234, #14145, #14308 ) ;
#7008=CARTESIAN_POINT ( 'NONE',  ( 21.09785597605720753, -14.04221034894631615, 105.7124997376166391 ) ) ;
#7049=CARTESIAN_POINT ( 'NONE',  ( 21.09785597605719332, 15.43591091851533115, 47.04930799450051637 ) ) ;
#7058=AXIS2_PLACEMENT_3D ( 'NONE', #16592, #16919, #9383 ) ;
#7059=DIRECTION ( 'NONE',  ( 0.000000000000000000, 0.000000000000000000, -1.000000000000000000 ) ) ;
#7083=DIRECTION ( 'NONE',  ( -1.000000000000000000, 0.000000000000000000, 0.000000000000000000 ) ) ;
#7088=CARTESIAN_POINT ( 'NONE',  ( 21.09785597605718976, 6.671061906060458568, 67.63280429334794519 ) ) ;
#7093=CARTESIAN_POINT ( 'NONE',  ( -17.37805493069431151, -13.74047052604243646, 90.91442668615566447 ) ) ;
#7096=DIRECTION ( 'NONE',  ( 0.000000000000000000, 1.000000000000000000, -0.000000000000000000 ) ) ;
#7098=CIRCLE ( 'NONE', #9181, 0.09999999999999766020 ) ;
#7119=ORIENTED_EDGE ( 'NONE', *, *, #23968, .T. ) ;
#7121=ORIENTED_EDGE ( 'NONE', *, *, #10321, .T. ) ;
#7137=DIRECTION ( 'NONE',  ( -0.000000000000000000, -1.000000000000000000, -0.000000000000000000 ) ) ;
#7159=EDGE_CURVE ( 'NONE', #26439, #16663, #23923, .T. ) ;
#7172=DIRECTION ( 'NONE',  ( -1.000000000000000000, 0.000000000000000000, -1.224646799147353207E-16 ) ) ;
#7214=ORIENTED_EDGE ( 'NONE', *, *, #29534, .F. ) ;
#7230=DIRECTION ( 'NONE',  ( 0.000000000000000000, 0.000000000000000000, -1.000000000000000000 ) ) ;
#7235=ORIENTED_EDGE ( 'NONE', *, *, #26667, .F. ) ;
#7237=CARTESIAN_POINT ( 'NONE',  ( 56.61384086331115384, -13.74047052604243646, 93.34357519277922677 ) ) ;
#7240=DIRECTION ( 'NONE',  ( 0.000000000000000000, 0.000000000000000000, -1.000000000000000000 ) ) ;
#7252=CIRCLE ( 'NONE', #7775, 12.78419020052701960 ) ;
#7255=FACE_OUTER_BOUND ( 'NONE', #6145, .T. ) ;
#7262=CARTESIAN_POINT ( 'NONE',  ( -29.43068460852080648, -13.74047052604243646, 17.87036105788322260 ) ) ;
#7301=DIRECTION ( 'NONE',  ( 0.000000000000000000, 0.000000000000000000, -1.000000000000000000 ) ) ;
#7317=DIRECTION ( 'NONE',  ( 0.000000000000000000, 0.000000000000000000, -1.000000000000000000 ) ) ;
#7328=DIRECTION ( 'NONE',  ( -0.000000000000000000, -1.000000000000000000, -0.000000000000000000 ) ) ;
#7361=AXIS2_PLACEMENT_3D ( 'NONE', #13661, #6262, #21178 ) ;
#7363=ORIENTED_EDGE ( 'NONE', *, *, #20777, .F. ) ;
#7384=CARTESIAN_POINT ( 'NONE',  ( 21.09785597605720042, -14.04221034894631615, 47.04930799450051637 ) ) ;
#7400=ORIENTED_EDGE ( 'NONE', *, *, #18447, .F. ) ;
#7408=VERTEX_POINT ( 'NONE', #17085 ) ;
#7424=AXIS2_PLACEMENT_3D ( 'NONE', #5020, #10272, #32268 ) ;
#7435=DIRECTION ( 'NONE',  ( 0.000000000000000000, 0.000000000000000000, -1.000000000000000000 ) ) ;
#7446=CARTESIAN_POINT ( 'NONE',  ( 21.09785597605720042, -16.63545420775220407, 47.04930799450051637 ) ) ;
#7489=VERTEX_POINT ( 'NONE', #17415 ) ;
#7491=FACE_OUTER_BOUND ( 'NONE', #13233, .T. ) ;
#7520=CIRCLE ( 'NONE', #15895, 0.6000000000000033085 ) ;
#7521=AXIS2_PLACEMENT_3D ( 'NONE', #6378, #5904, #6213 ) ;
#7594=( NAMED_UNIT ( * ) PLANE_ANGLE_UNIT ( ) SI_UNIT ( $, .RADIAN. ) );
#7614=AXIS2_PLACEMENT_3D ( 'NONE', #10300, #30318, #22101 ) ;
#7662=ORIENTED_EDGE ( 'NONE', *, *, #29534, .T. ) ;
#7707=DIRECTION ( 'NONE',  ( 0.000000000000000000, 0.000000000000000000, -1.000000000000000000 ) ) ;
#7718=CIRCLE ( 'NONE', #26046, 12.73401709983438401 ) ;
#7742=DIRECTION ( 'NONE',  ( 1.000000000000000000, 0.000000000000000000, -1.224646799147353207E-16 ) ) ;
#7745=AXIS2_PLACEMENT_3D ( 'NONE', #7780, #17781, #22870 ) ;
#7760=EDGE_CURVE ( 'NONE', #20587, #1157, #11326, .T. ) ;
#7775=AXIS2_PLACEMENT_3D ( 'NONE', #20885, #28450, #25974 ) ;
#7780=CARTESIAN_POINT ( 'NONE',  ( 21.09785597605720042, -13.87844638871996850, 47.04930799450051637 ) ) ;
#7794=DIRECTION ( 'NONE',  ( 0.000000000000000000, 1.000000000000000000, -0.000000000000000000 ) ) ;
#7866=ADVANCED_FACE ( 'NONE', ( #29863 ), #12380, .T. ) ;
#7869=LINE ( 'NONE', #20653, #30674 ) ;
#7938=VECTOR ( 'NONE', #17287, 1000.000000000000000 ) ;
#7943=CONICAL_SURFACE ( 'NONE', #7424, 55.69429210806286079, 1.269872874662818729 ) ;
#7955=AXIS2_PLACEMENT_3D ( 'NONE', #32135, #31963, #4389 ) ;
#7960=CARTESIAN_POINT ( 'NONE',  ( 21.09785597605720042, -14.04221034894631615, -11.81388374861560386 ) ) ;
#7968=CARTESIAN_POINT ( 'NONE',  ( 21.09785597605720042, -52.14605111273580462, -31.45069200549948363 ) ) ;
#7969=ORIENTED_EDGE ( 'NONE', *, *, #31621, .T. ) ;
#7977=CARTESIAN_POINT ( 'NONE',  ( 21.09785597605719332, 6.717634499306958773, 47.04930799450051637 ) ) ;
#8006=TOROIDAL_SURFACE ( 'NONE', #660, 13.48414152717812797, 1.000000000001010525 ) ;
#8013=LINE ( 'NONE', #20471, #32416 ) ;
#8028=AXIS2_PLACEMENT_3D ( 'NONE', #17543, #14928, #17379 ) ;
#8042=ORIENTED_EDGE ( 'NONE', *, *, #26257, .F. ) ;
#8049=ORIENTED_EDGE ( 'NONE', *, *, #24115, .T. ) ;
#8080=FACE_OUTER_BOUND ( 'NONE', #24110, .T. ) ;
#8083=EDGE_CURVE ( 'NONE', #16663, #11145, #28638, .T. ) ;
#8087=CARTESIAN_POINT ( 'NONE',  ( 55.14312657641617221, -13.30632128221581389, 91.42653303877501969 ) ) ;
#8115=AXIS2_PLACEMENT_3D ( 'NONE', #4467, #3531, #8472 ) ;
#8120=CONICAL_SURFACE ( 'NONE', #4984, 55.68770647617149905, 0.3009234521320683364 ) ;
#8121=AXIS2_PLACEMENT_3D ( 'NONE', #32131, #5376, #14896 ) ;
#8137=ADVANCED_FACE ( 'NONE', ( #9102 ), #24029, .T. ) ;
#8141=ORIENTED_EDGE ( 'NONE', *, *, #1070, .T. ) ;
#8143=CONICAL_SURFACE ( 'NONE', #2881, 20.38082872909741994, 1.021642509542357802 ) ;
#8146=CIRCLE ( 'NONE', #25451, 69.99901951359278485 ) ;
#8172=AXIS2_PLACEMENT_3D ( 'NONE', #6286, #1354, #5977 ) ;
#8195=ORIENTED_EDGE ( 'NONE', *, *, #19559, .F. ) ;
#8201=DIRECTION ( 'NONE',  ( -0.000000000000000000, -1.000000000000000000, -0.000000000000000000 ) ) ;
#8226=CARTESIAN_POINT ( 'NONE',  ( -31.86441722936940479, -13.30632128221581212, 65.03308317646940395 ) ) ;
#8256=ORIENTED_EDGE ( 'NONE', *, *, #19061, .T. ) ;
#8279=DIRECTION ( 'NONE',  ( -0.000000000000000000, -1.000000000000000000, -0.000000000000000000 ) ) ;
#8285=DIRECTION ( 'NONE',  ( 0.000000000000000000, 0.000000000000000000, -1.000000000000000000 ) ) ;
#8293=ORIENTED_EDGE ( 'NONE', *, *, #5463, .F. ) ;
#8297=AXIS2_PLACEMENT_3D ( 'NONE', #20636, #30658, #28189 ) ;
#8299=LINE ( 'NONE', #10448, #6186 ) ;
#8310=ORIENTED_EDGE ( 'NONE', *, *, #9477, .T. ) ;
#8331=AXIS2_PLACEMENT_3D ( 'NONE', #27338, #29974, #8285 ) ;
#8338=AXIS2_PLACEMENT_3D ( 'NONE', #18760, #31588, #24021 ) ;
#8361=DIRECTION ( 'NONE',  ( 0.000000000000000000, 1.000000000000000000, -0.000000000000000000 ) ) ;
#8372=CONICAL_SURFACE ( 'NONE', #1540, 55.68770647617149905, 0.3009234521320683364 ) ;
#8377=LINE ( 'NONE', #18377, #23300 ) ;
#8386=EDGE_LOOP ( 'NONE', ( #32476, #23442, #3540, #3009 ) ) ;
#8400=CIRCLE ( 'NONE', #26214, 58.66319174311612272 ) ;
#8403=ORIENTED_EDGE ( 'NONE', *, *, #24893, .T. ) ;
#8435=CARTESIAN_POINT ( 'NONE',  ( 21.09785597605719332, 17.36451738380053555, 59.73344952167762756 ) ) ;
#8439=CONICAL_SURFACE ( 'NONE', #22037, 58.09216821878680292, 1.269872874662833384 ) ;
#8453=ORIENTED_EDGE ( 'NONE', *, *, #4545, .F. ) ;
#8462=ADVANCED_BREP_SHAPE_REPRESENTATION ( '', ( #12396, #8172 ), #824 ) ;
#8472=DIRECTION ( 'NONE',  ( 0.000000000000000000, 0.000000000000000000, -1.000000000000000000 ) ) ;
#8516=ORIENTED_EDGE ( 'NONE', *, *, #27659, .F. ) ;
#8530=DIRECTION ( 'NONE',  ( 0.000000000000000000, 0.000000000000000000, -1.000000000000000000 ) ) ;
#8533=ORIENTED_EDGE ( 'NONE', *, *, #17749, .T. ) ;
#8553=DIRECTION ( 'NONE',  ( -0.000000000000000000, -1.000000000000000000, -0.000000000000000000 ) ) ;
#8572=ADVANCED_FACE ( 'NONE', ( #16282 ), #26959, .F. ) ;
#8594=ADVANCED_FACE ( 'NONE', ( #1672 ), #2320, .T. ) ;
#8603=CARTESIAN_POINT ( 'NONE',  ( 21.09785597605719332, 7.237299147902269247, 47.04930799450051637 ) ) ;
#8635=CARTESIAN_POINT ( 'NONE',  ( 21.09785597605720042, -16.03545420775220265, 47.04930799450051637 ) ) ;
#8639=EDGE_CURVE ( 'NONE', #26708, #529, #17017, .T. ) ;
#8648=DIRECTION ( 'NONE',  ( -0.000000000000000000, -1.000000000000000000, -0.000000000000000000 ) ) ;
#8655=VERTEX_POINT ( 'NONE', #7088 ) ;
#8665=EDGE_CURVE ( 'NONE', #27949, #20946, #5486, .T. ) ;
#8684=DIRECTION ( 'NONE',  ( 0.000000000000000000, 0.000000000000000000, -1.000000000000000000 ) ) ;
#8710=ORIENTED_EDGE ( 'NONE', *, *, #5908, .F. ) ;
#8717=CARTESIAN_POINT ( 'NONE',  ( 35.56915586375613003, -13.30632128221580857, 101.0770789316965903 ) ) ;
#8764=VERTEX_POINT ( 'NONE', #15927 ) ;
#8770=CARTESIAN_POINT ( 'NONE',  ( 21.09785597605720753, -13.37218737171702543, 102.7370144706720225 ) ) ;
#8838=CARTESIAN_POINT ( 'NONE',  ( 21.09785597605719332, 7.264443105416139801, 47.04930799450051637 ) ) ;
#8868=CARTESIAN_POINT ( 'NONE',  ( 21.09785597605719332, 77.37245976740706510, 47.04930799450051637 ) ) ;
#8883=DIRECTION ( 'NONE',  ( -0.000000000000000000, -1.000000000000000000, -0.000000000000000000 ) ) ;
#8906=CARTESIAN_POINT ( 'NONE',  ( 21.09785597605720042, -13.88867167006704939, 47.04930799450051637 ) ) ;
#8916=DIRECTION ( 'NONE',  ( 0.000000000000000000, 1.000000000000000000, -0.000000000000000000 ) ) ;
#8921=DIRECTION ( 'NONE',  ( 0.000000000000000000, 0.000000000000000000, -1.000000000000000000 ) ) ;
#8926=ORIENTED_EDGE ( 'NONE', *, *, #2404, .F. ) ;
#8931=ADVANCED_FACE ( 'NONE', ( #9353 ), #16480, .T. ) ;
#8979=VECTOR ( 'NONE', #18634, 1000.000000000000341 ) ;
#8981=DIRECTION ( 'NONE',  ( -0.000000000000000000, -1.000000000000000000, -0.000000000000000000 ) ) ;
#8984=CARTESIAN_POINT ( 'NONE',  ( 21.09785597605720042, -13.88867167006704939, 105.7507399849467333 ) ) ;
#8998=FACE_OUTER_BOUND ( 'NONE', #25285, .T. ) ;
#9019=CYLINDRICAL_SURFACE ( 'NONE', #31196, 12.48414152717711900 ) ;
#9028=EDGE_CURVE ( 'NONE', #17607, #21751, #20193, .T. ) ;
#9031=EDGE_CURVE ( 'NONE', #26992, #3864, #27537, .T. ) ;
#9038=CARTESIAN_POINT ( 'NONE',  ( 39.08163115802606313, -13.30632128221581034, -5.912965210926095061 ) ) ;
#9046=CARTESIAN_POINT ( 'NONE',  ( 76.34803497562472785, -13.74047052604243468, 28.28865559504965077 ) ) ;
#9053=CIRCLE ( 'NONE', #13274, 1.000000000000000888 ) ;
#9085=ORIENTED_EDGE ( 'NONE', *, *, #14998, .F. ) ;
#9086=DIRECTION ( 'NONE',  ( 0.000000000000000000, 0.000000000000000000, -1.000000000000000000 ) ) ;
#9093=EDGE_LOOP ( 'NONE', ( #17876, #3245, #7363, #32021 ) ) ;
#9102=FACE_OUTER_BOUND ( 'NONE', #32353, .T. ) ;
#9181=AXIS2_PLACEMENT_3D ( 'NONE', #27075, #12414, #21975 ) ;
#9197=FACE_OUTER_BOUND ( 'NONE', #9372, .T. ) ;
#9202=VERTEX_POINT ( 'NONE', #307 ) ;
#9208=ORIENTED_EDGE ( 'NONE', *, *, #5577, .F. ) ;
#9210=CARTESIAN_POINT ( 'NONE',  ( 46.89984767728657999, -13.74047052604243291, -5.284252768999646577 ) ) ;
#9222=ADVANCED_FACE ( 'NONE', ( #15897 ), #9707, .T. ) ;
#9228=DIRECTION ( 'NONE',  ( -0.000000000000000000, -1.000000000000000000, -0.000000000000000000 ) ) ;
#9235=CARTESIAN_POINT ( 'NONE',  ( 17.28711060612851469, -13.74047052604243468, 105.2732083934160840 ) ) ;
#9258=EDGE_CURVE ( 'NONE', #28679, #10039, #7869, .T. ) ;
#9306=DIRECTION ( 'NONE',  ( 0.000000000000000000, 0.000000000000000000, -1.000000000000000000 ) ) ;
#9312=ORIENTED_EDGE ( 'NONE', *, *, #5943, .F. ) ;
#9353=FACE_OUTER_BOUND ( 'NONE', #23955, .T. ) ;
#9358=ORIENTED_EDGE ( 'NONE', *, *, #10555, .T. ) ;
#9362=CARTESIAN_POINT ( 'NONE',  ( 21.09785597605718976, -13.68121847681060643, -10.98357976667645808 ) ) ;
#9366=CARTESIAN_POINT ( 'NONE',  ( 63.14652337230383949, -13.30632128221581212, 10.16668169048476855 ) ) ;
#9367=CARTESIAN_POINT ( 'NONE',  ( 21.09785597605720042, -16.93545420775220123, -31.45069200549948363 ) ) ;
#9372=EDGE_LOOP ( 'NONE', ( #25606, #23426, #55, #2646 ) ) ;
#9383=DIRECTION ( 'NONE',  ( 0.000000000000000000, 0.000000000000000000, -1.000000000000000000 ) ) ;
#9396=CARTESIAN_POINT ( 'NONE',  ( -36.75072804420383932, -13.74047052604243646, 39.42791148283190950 ) ) ;
#9398=ADVANCED_FACE ( 'NONE', ( #28851 ), #24930, .T. ) ;
#9426=EDGE_CURVE ( 'NONE', #30184, #529, #12357, .T. ) ;
#9447=CARTESIAN_POINT ( 'NONE',  ( 21.09785597605719332, 77.37245976740706510, -36.90550222348115028 ) ) ;
#9462=VERTEX_POINT ( 'NONE', #7008 ) ;
#9477=EDGE_CURVE ( 'NONE', #14445, #28679, #2399, .T. ) ;
#9480=ORIENTED_EDGE ( 'NONE', *, *, #22080, .T. ) ;
#9498=FACE_OUTER_BOUND ( 'NONE', #31590, .T. ) ;
#9521=ORIENTED_EDGE ( 'NONE', *, *, #2484, .F. ) ;
#9542=CARTESIAN_POINT ( 'NONE',  ( 21.09785597605719332, -13.74048473023143835, 105.2732083928529221 ) ) ;
#9545=FACE_OUTER_BOUND ( 'NONE', #14610, .T. ) ;
#9546=DIRECTION ( 'NONE',  ( 1.000000000000000000, 0.000000000000000000, 0.000000000000000000 ) ) ;
#9560=CARTESIAN_POINT ( 'NONE',  ( 21.09785597605720042, -14.04221034894631615, 47.04930799450051637 ) ) ;
#9562=CARTESIAN_POINT ( 'NONE',  ( -4.704135725172235105, -13.74047052604243646, -5.284252768999630590 ) ) ;
#9583=ADVANCED_FACE ( 'NONE', ( #17335 ), #29826, .T. ) ;
#9586=FACE_OUTER_BOUND ( 'NONE', #11186, .T. ) ;
#9658=CARTESIAN_POINT ( 'NONE',  ( 1.839586350524081038, 7.881678200673685630, 47.04930799450051637 ) ) ;
#9682=VERTEX_POINT ( 'NONE', #30480 ) ;
#9686=ORIENTED_EDGE ( 'NONE', *, *, #5361, .F. ) ;
#9707=CONICAL_SURFACE ( 'NONE', #27013, 58.09216821878680292, 1.269872874662833384 ) ;
#9709=AXIS2_PLACEMENT_3D ( 'NONE', #78, #7794, #25351 ) ;
#9755=LINE ( 'NONE', #29776, #7938 ) ;
#9760=EDGE_CURVE ( 'NONE', #20704, #5958, #22247, .T. ) ;
#9803=EDGE_LOOP ( 'NONE', ( #20825, #11661 ) ) ;
#9817=ADVANCED_FACE ( 'NONE', ( #15858 ), #28547, .F. ) ;
#9822=CARTESIAN_POINT ( 'NONE',  ( 21.09785597605720042, -52.14605111273580462, 47.04930799450051637 ) ) ;
#9847=CARTESIAN_POINT ( 'NONE',  ( 21.09785597605720042, -17.03545420775220265, 47.04930799450051637 ) ) ;
#9848=CARTESIAN_POINT ( 'NONE',  ( 21.09785597605720042, -13.98292989133646103, -11.62287111200335055 ) ) ;
#9849=CIRCLE ( 'NONE', #12483, 12.98419020052701889 ) ;
#9888=( LENGTH_UNIT ( ) NAMED_UNIT ( * ) SI_UNIT ( .MILLI., .METRE. ) );
#9900=DIRECTION ( 'NONE',  ( 1.000000000000000000, 0.000000000000000000, 0.000000000000000000 ) ) ;
#9927=CARTESIAN_POINT ( 'NONE',  ( 40.35612560159030693, 7.881678200673685630, 47.04930799450051637 ) ) ;
#9928=DIRECTION ( 'NONE',  ( 0.000000000000000000, 0.000000000000000000, -1.000000000000000000 ) ) ;
#9934=DIRECTION ( 'NONE',  ( 0.000000000000000000, 0.000000000000000000, -1.000000000000000000 ) ) ;
#9942=ADVANCED_FACE ( 'NONE', ( #29917 ), #8143, .T. ) ;
#9954=DIRECTION ( 'NONE',  ( 0.000000000000000000, 0.000000000000000000, -1.000000000000000000 ) ) ;
#9982=ORIENTED_EDGE ( 'NONE', *, *, #31237, .T. ) ;
#10002=AXIS2_PLACEMENT_3D ( 'NONE', #15751, #28881, #8530 ) ;
#10006=CARTESIAN_POINT ( 'NONE',  ( 21.09785597605719332, 7.237299147902269247, 47.04930799450051637 ) ) ;
#10010=EDGE_CURVE ( 'NONE', #24256, #14178, #19094, .T. ) ;
#10014=AXIS2_PLACEMENT_3D ( 'NONE', #27193, #17176, #29336 ) ;
#10016=ORIENTED_EDGE ( 'NONE', *, *, #9031, .F. ) ;
#10036=DIRECTION ( 'NONE',  ( 0.000000000000000000, 1.000000000000000000, -0.000000000000000000 ) ) ;
#10039=VERTEX_POINT ( 'NONE', #5771 ) ;
#10050=DIRECTION ( 'NONE',  ( 0.000000000000000000, 0.000000000000000000, -1.000000000000000000 ) ) ;
#10052=ADVANCED_FACE ( 'NONE', ( #3457 ), #25927, .F. ) ;
#10097=EDGE_CURVE ( 'NONE', #23467, #30184, #11280, .T. ) ;
#10107=DIRECTION ( 'NONE',  ( 0.000000000000000000, 0.000000000000000000, -1.000000000000000000 ) ) ;
#10113=DIRECTION ( 'NONE',  ( 0.000000000000000000, 0.000000000000000000, -1.000000000000000000 ) ) ;
#10114=CIRCLE ( 'NONE', #13755, 5.099019513592789821 ) ;
#10120=TOROIDAL_SURFACE ( 'NONE', #14309, 20.27643559902816861, 0.2000000000000001499 ) ;
#10231=EDGE_CURVE ( 'NONE', #15416, #13009, #29096, .T. ) ;
#10234=LINE ( 'NONE', #13018, #24637 ) ;
#10240=ADVANCED_FACE ( 'NONE', ( #16410 ), #21489, .T. ) ;
#10245=ADVANCED_FACE ( 'NONE', ( #9197 ), #24288, .F. ) ;
#10272=DIRECTION ( 'NONE',  ( -0.000000000000000000, -1.000000000000000000, -0.000000000000000000 ) ) ;
#10285=EDGE_CURVE ( 'NONE', #11145, #16663, #4407, .T. ) ;
#10287=EDGE_CURVE ( 'NONE', #8655, #1157, #4999, .T. ) ;
#10300=CARTESIAN_POINT ( 'NONE',  ( 21.09785597605720042, -14.24176827912842391, 47.04930799450051637 ) ) ;
#10303=ORIENTED_EDGE ( 'NONE', *, *, #4339, .T. ) ;
#10321=EDGE_CURVE ( 'NONE', #13009, #20809, #7098, .T. ) ;
#10347=ORIENTED_EDGE ( 'NONE', *, *, #20239, .F. ) ;
#10369=CARTESIAN_POINT ( 'NONE',  ( 21.09785597605720042, -16.73545420775220194, 47.04930799450051637 ) ) ;
#10409=EDGE_CURVE ( 'NONE', #31613, #29876, #3414, .T. ) ;
#10432=CARTESIAN_POINT ( 'NONE',  ( 21.09785597605720042, -13.87844638871996850, -12.39237876099712210 ) ) ;
#10440=TOROIDAL_SURFACE ( 'NONE', #4135, 58.86319174311611846, 0.1999999999999984290 ) ;
#10448=CARTESIAN_POINT ( 'NONE',  ( 21.09785597605720753, -13.98292989133646103, -11.62287111200335055 ) ) ;
#10463=ORIENTED_EDGE ( 'NONE', *, *, #10010, .F. ) ;
#10465=AXIS2_PLACEMENT_3D ( 'NONE', #28785, #16467, #8921 ) ;
#10477=AXIS2_PLACEMENT_3D ( 'NONE', #5835, #13064, #30940 ) ;
#10492=FACE_OUTER_BOUND ( 'NONE', #23481, .T. ) ;
#10540=DIRECTION ( 'NONE',  ( 0.000000000000000000, 0.000000000000000000, -1.000000000000000000 ) ) ;
#10555=EDGE_CURVE ( 'NONE', #18375, #28679, #2909, .T. ) ;
#10588=FACE_OUTER_BOUND ( 'NONE', #26435, .T. ) ;
#10611=ORIENTED_EDGE ( 'NONE', *, *, #18447, .T. ) ;
#10658=ORIENTED_EDGE ( 'NONE', *, *, #4905, .F. ) ;
#10682=DIRECTION ( 'NONE',  ( 0.000000000000000000, 0.000000000000000000, -1.000000000000000000 ) ) ;
#10693=EDGE_LOOP ( 'NONE', ( #29968, #5521, #5395, #28759 ) ) ;
#10701=DIRECTION ( 'NONE',  ( -0.000000000000000000, -1.000000000000000000, -0.000000000000000000 ) ) ;
#10703=CARTESIAN_POINT ( 'NONE',  ( -15.78477032795854207, -13.30632128221581389, 89.09797539074716610 ) ) ;
#10714=ORIENTED_EDGE ( 'NONE', *, *, #12573, .F. ) ;
#10722=CARTESIAN_POINT ( 'NONE',  ( 21.09785597605719332, 7.094379510609982731, 47.04930799450051637 ) ) ;
#10743=CARTESIAN_POINT ( 'NONE',  ( 21.09785597605719332, 14.77310068074637961, 47.04930799450051637 ) ) ;
#10752=AXIS2_PLACEMENT_3D ( 'NONE', #15113, #12501, #12669 ) ;
#10756=CARTESIAN_POINT ( 'NONE',  ( 21.09785597605720753, -14.04221034894631615, 105.9124997376166277 ) ) ;
#10761=ORIENTED_EDGE ( 'NONE', *, *, #25610, .T. ) ;
#10763=DIRECTION ( 'NONE',  ( 0.000000000000000000, 0.000000000000000000, -1.000000000000000000 ) ) ;
#10776=DIRECTION ( 'NONE',  ( 0.000000000000000000, 0.000000000000000000, -1.000000000000000000 ) ) ;
#10795=DIRECTION ( 'NONE',  ( -0.000000000000000000, -1.000000000000000000, -0.000000000000000000 ) ) ;
#10855=CARTESIAN_POINT ( 'NONE',  ( 21.09785597605719687, -13.30631372918550959, -8.763520691563154941 ) ) ;
#10870=CARTESIAN_POINT ( 'NONE',  ( 76.55093444394999835, -13.30632128221581567, 54.35510304470366094 ) ) ;
#10876=DIRECTION ( 'NONE',  ( -1.000000000000000000, 0.000000000000000000, 0.000000000000000000 ) ) ;
#10879=DIRECTION ( 'NONE',  ( 0.000000000000000000, 0.000000000000000000, -1.000000000000000000 ) ) ;
#10926=AXIS2_PLACEMENT_3D ( 'NONE', #5701, #25727, #3233 ) ;
#10930=ORIENTED_EDGE ( 'NONE', *, *, #25318, .F. ) ;
#10948=FACE_OUTER_BOUND ( 'NONE', #22242, .T. ) ;
#10954=EDGE_CURVE ( 'NONE', #23177, #15932, #13734, .T. ) ;
#10988=EDGE_CURVE ( 'NONE', #20946, #14445, #15229, .T. ) ;
#10998=DIRECTION ( 'NONE',  ( 0.000000000000000000, 0.000000000000000000, -1.000000000000000000 ) ) ;
#11000=AXIS2_PLACEMENT_3D ( 'NONE', #11551, #28957, #31099 ) ;
#11014=CARTESIAN_POINT ( 'NONE',  ( -34.35522249183560461, -13.30632128221581212, 54.35510304470367515 ) ) ;
#11016=FACE_OUTER_BOUND ( 'NONE', #6637, .T. ) ;
#11052=AXIS2_PLACEMENT_3D ( 'NONE', #17672, #5212, #23089 ) ;
#11060=VECTOR ( 'NONE', #8279, 1000.000000000000000 ) ;
#11072=DIRECTION ( 'NONE',  ( 0.000000000000000000, 0.000000000000000000, -1.000000000000000000 ) ) ;
#11078=VERTEX_POINT ( 'NONE', #16820 ) ;
#11094=EDGE_CURVE ( 'NONE', #15585, #11769, #20469, .T. ) ;
#11143=VERTEX_POINT ( 'NONE', #11850 ) ;
#11145=VERTEX_POINT ( 'NONE', #21845 ) ;
#11148=DIRECTION ( 'NONE',  ( 0.000000000000000000, 0.000000000000000000, -1.000000000000000000 ) ) ;
#11157=EDGE_LOOP ( 'NONE', ( #12436, #18311 ) ) ;
#11175=DIRECTION ( 'NONE',  ( 1.000000000000000000, 0.000000000000000000, 0.000000000000000000 ) ) ;
#11186=EDGE_LOOP ( 'NONE', ( #24099, #12792, #20130, #24245 ) ) ;
#11246=DIRECTION ( 'NONE',  ( -0.000000000000000000, -1.000000000000000000, -0.000000000000000000 ) ) ;
#11260=DIRECTION ( 'NONE',  ( 0.000000000000000000, 0.000000000000000000, -1.000000000000000000 ) ) ;
#11280=CIRCLE ( 'NONE', #15472, 12.73401709983438401 ) ;
#11281=AXIS2_PLACEMENT_3D ( 'NONE', #22064, #19106, #24702 ) ;
#11292=CARTESIAN_POINT ( 'NONE',  ( 21.09785597605719332, 15.24673779880127178, 47.04930799450051637 ) ) ;
#11297=CIRCLE ( 'NONE', #6074, 58.67217910650386870 ) ;
#11308=DIRECTION ( 'NONE',  ( 0.000000000000000000, 1.000000000000000000, -0.000000000000000000 ) ) ;
#11326=LINE ( 'NONE', #13792, #2918 ) ;
#11330=CARTESIAN_POINT ( 'NONE',  ( 13.79206092585405230, -13.30632128221581212, 102.5023864623932894 ) ) ;
#11331=DIRECTION ( 'NONE',  ( 0.000000000000000000, 0.000000000000000000, -1.000000000000000000 ) ) ;
#11333=VERTEX_POINT ( 'NONE', #22097 ) ;
#11339=EDGE_LOOP ( 'NONE', ( #7214, #24769, #31421, #202 ) ) ;
#11347=ORIENTED_EDGE ( 'NONE', *, *, #25214, .F. ) ;
#11348=CARTESIAN_POINT ( 'NONE',  ( 50.27680291267449775, -13.74047052604243468, -3.479232590077480758 ) ) ;
#11351=FACE_OUTER_BOUND ( 'NONE', #18688, .T. ) ;
#11379=EDGE_CURVE ( 'NONE', #14004, #30037, #1624, .T. ) ;
#11387=CIRCLE ( 'NONE', #29736, 19.45967690998103805 ) ;
#11497=CARTESIAN_POINT ( 'NONE',  ( 24.75079866426201392, -13.30632128221581034, -8.763545028782029789 ) ) ;
#11548=CIRCLE ( 'NONE', #27644, 36.51080762834750715 ) ;
#11551=CARTESIAN_POINT ( 'NONE',  ( 21.09785597605720042, -16.03545420775219910, -17.45069200549948718 ) ) ;
#11563=MECHANICAL_DESIGN_GEOMETRIC_PRESENTATION_REPRESENTATION('',(#13150),#6858);
#11568=DIRECTION ( 'NONE',  ( 0.000000000000000000, 0.000000000000000000, -1.000000000000000000 ) ) ;
#11613=DIRECTION ( 'NONE',  ( 0.000000000000000000, 0.000000000000000000, -1.000000000000000000 ) ) ;
#11661=ORIENTED_EDGE ( 'NONE', *, *, #10010, .T. ) ;
#11672=DIRECTION ( 'NONE',  ( -0.000000000000000000, -1.000000000000000000, -0.000000000000000000 ) ) ;
#11681=DIRECTION ( 'NONE',  ( -0.000000000000000000, -1.000000000000000000, -0.000000000000000000 ) ) ;
#11683=ADVANCED_FACE ( 'NONE', ( #16643 ), #28887, .T. ) ;
#11690=DIRECTION ( 'NONE',  ( 0.000000000000000000, 0.000000000000000000, -1.000000000000000000 ) ) ;
#11769=VERTEX_POINT ( 'NONE', #9927 ) ;
#11796=AXIS2_PLACEMENT_3D ( 'NONE', #16853, #7172, #19798 ) ;
#11817=AXIS2_PLACEMENT_3D ( 'NONE', #24700, #14858, #9928 ) ;
#11830=DIRECTION ( 'NONE',  ( 0.000000000000000000, 1.000000000000000000, -0.000000000000000000 ) ) ;
#11834=CARTESIAN_POINT ( 'NONE',  ( 65.47508102033168598, -13.30632128221580857, 13.00403739414153570 ) ) ;
#11849=DIRECTION ( 'NONE',  ( -1.000000000000000000, 0.000000000000000000, 0.000000000000000000 ) ) ;
#11850=CARTESIAN_POINT ( 'NONE',  ( 21.09785597605719332, 17.36451738380053555, 34.26511779397349500 ) ) ;
#11885=VERTEX_POINT ( 'NONE', #8435 ) ;
#11895=CARTESIAN_POINT ( 'NONE',  ( 21.09785597605720042, -16.03545420775220265, 47.04930799450051637 ) ) ;
#11904=CARTESIAN_POINT ( 'NONE',  ( 21.09785597605721108, -16.93545420775220478, 125.4493079945005150 ) ) ;
#11928=EDGE_CURVE ( 'NONE', #25082, #16711, #15275, .T. ) ;
#11967=CARTESIAN_POINT ( 'NONE',  ( 21.09785597605719332, 38.31023907818019580, 47.04930799450051637 ) ) ;
#11992=EDGE_LOOP ( 'NONE', ( #3784, #24790, #4331, #24293 ) ) ;
#11998=CARTESIAN_POINT ( 'NONE',  ( 36.19429842010746512, -13.74047052604243646, 103.4110129320798563 ) ) ;
#12006=ADVANCED_FACE ( 'NONE', ( #31566 ), #5322, .T. ) ;
#12013=DIRECTION ( 'NONE',  ( 0.000000000000000000, 1.000000000000000000, -0.000000000000000000 ) ) ;
#12014=DIRECTION ( 'NONE',  ( -0.000000000000000000, -1.000000000000000000, -0.000000000000000000 ) ) ;
#12042=EDGE_CURVE ( 'NONE', #24243, #29876, #19455, .T. ) ;
#12061=EDGE_CURVE ( 'NONE', #24037, #8764, #13687, .T. ) ;
#12126=AXIS2_PLACEMENT_3D ( 'NONE', #12220, #24513, #16632 ) ;
#12136=AXIS2_PLACEMENT_3D ( 'NONE', #8906, #6453, #4141 ) ;
#12148=ORIENTED_EDGE ( 'NONE', *, *, #32211, .F. ) ;
#12193=AXIS2_PLACEMENT_3D ( 'NONE', #30559, #18538, #834 ) ;
#12217=ORIENTED_EDGE ( 'NONE', *, *, #16733, .T. ) ;
#12220=CARTESIAN_POINT ( 'NONE',  ( 21.09785597605720042, -14.03534765547855656, 47.04930799450051637 ) ) ;
#12223=CIRCLE ( 'NONE', #22168, 12.98419020052702599 ) ;
#12237=DIRECTION ( 'NONE',  ( 0.000000000000000000, 0.000000000000000000, -1.000000000000000000 ) ) ;
#12298=DIRECTION ( 'NONE',  ( -1.044582700994767690E-16, 0.5219656503457801300, 0.8529665057076430967 ) ) ;
#12302=FACE_OUTER_BOUND ( 'NONE', #31221, .T. ) ;
#12310=CARTESIAN_POINT ( 'NONE',  ( 21.09785597605720042, -16.03545420775219910, 47.04930799450051637 ) ) ;
#12347=DIRECTION ( 'NONE',  ( -0.000000000000000000, -1.000000000000000000, -0.000000000000000000 ) ) ;
#12357=CIRCLE ( 'NONE', #28077, 94.94530576803560962 ) ;
#12376=ORIENTED_EDGE ( 'NONE', *, *, #14166, .T. ) ;
#12380=TOROIDAL_SURFACE ( 'NONE', #15001, 12.78419020052701960, 0.2000000000000000944 ) ;
#12396=MANIFOLD_SOLID_BREP ( 'Stock-MAT-060-1', #32042 ) ;
#12414=DIRECTION ( 'NONE',  ( -1.000000000000000000, 0.000000000000000000, 0.000000000000000000 ) ) ;
#12436=ORIENTED_EDGE ( 'NONE', *, *, #24115, .F. ) ;
#12469=ORIENTED_EDGE ( 'NONE', *, *, #10988, .T. ) ;
#12470=DIRECTION ( 'NONE',  ( 0.000000000000000000, 0.000000000000000000, -1.000000000000000000 ) ) ;
#12483=AXIS2_PLACEMENT_3D ( 'NONE', #15071, #19986, #4560 ) ;
#12501=DIRECTION ( 'NONE',  ( 0.000000000000000000, 1.000000000000000000, -0.000000000000000000 ) ) ;
#12550=ORIENTED_EDGE ( 'NONE', *, *, #12042, .T. ) ;
#12552=CARTESIAN_POINT ( 'NONE',  ( 21.09785597605720753, -13.68834655544033652, 102.7436001025633772 ) ) ;
#12573=EDGE_CURVE ( 'NONE', #28679, #14445, #26787, .T. ) ;
#12577=VERTEX_POINT ( 'NONE', #14703 ) ;
#12585=EDGE_CURVE ( 'NONE', #20587, #20020, #3196, .T. ) ;
#12605=DIRECTION ( 'NONE',  ( 1.000000000000000000, 0.000000000000000000, 0.000000000000000000 ) ) ;
#12608=AXIS2_PLACEMENT_3D ( 'NONE', #3118, #10701, #26089 ) ;
#12613=CIRCLE ( 'NONE', #30950, 58.70143199044622406 ) ;
#12621=EDGE_CURVE ( 'NONE', #9462, #7489, #27839, .T. ) ;
#12622=FACE_OUTER_BOUND ( 'NONE', #23338, .T. ) ;
#12628=EDGE_CURVE ( 'NONE', #31146, #26439, #25673, .T. ) ;
#12630=CIRCLE ( 'NONE', #4223, 0.1999999999999970690 ) ;
#12646=EDGE_LOOP ( 'NONE', ( #22121, #18106, #22544, #32477 ) ) ;
#12655=ORIENTED_EDGE ( 'NONE', *, *, #20082, .T. ) ;
#12669=DIRECTION ( 'NONE',  ( 0.000000000000000000, 0.000000000000000000, -1.000000000000000000 ) ) ;
#12712=CARTESIAN_POINT ( 'NONE',  ( 21.09785597605720042, -16.93545420775220123, 47.04930799450051637 ) ) ;
#12740=CARTESIAN_POINT ( 'NONE',  ( 21.09785597605719332, 6.547041198165487685, 47.04930799450051637 ) ) ;
#12751=CARTESIAN_POINT ( 'NONE',  ( 21.09785597605719332, 17.16451738380053627, 47.04930799450051637 ) ) ;
#12766=ORIENTED_EDGE ( 'NONE', *, *, #25214, .T. ) ;
#12767=DIRECTION ( 'NONE',  ( -0.000000000000000000, -1.000000000000000000, -0.000000000000000000 ) ) ;
#12771=CARTESIAN_POINT ( 'NONE',  ( 21.09785597605719332, 17.16451738380053627, 47.04930799450051637 ) ) ;
#12787=ORIENTED_EDGE ( 'NONE', *, *, #4615, .T. ) ;
#12792=ORIENTED_EDGE ( 'NONE', *, *, #22565, .T. ) ;
#12796=ORIENTED_EDGE ( 'NONE', *, *, #17146, .T. ) ;
#12800=DIRECTION ( 'NONE',  ( 0.000000000000000000, 0.000000000000000000, 1.000000000000000000 ) ) ;
#12838=CIRCLE ( 'NONE', #16996, 19.21451602543517367 ) ;
#12845=DIRECTION ( 'NONE',  ( 0.000000000000000000, 0.000000000000000000, -1.000000000000000000 ) ) ;
#12860=CARTESIAN_POINT ( 'NONE',  ( 21.09785597605719332, 34.11266481626051217, 60.03349819502754059 ) ) ;
#12870=DIRECTION ( 'NONE',  ( 0.000000000000000000, 0.000000000000000000, 1.000000000000000000 ) ) ;
#12893=DIRECTION ( 'NONE',  ( 0.000000000000000000, 0.000000000000000000, 1.000000000000000000 ) ) ;
#12906=DIRECTION ( 'NONE',  ( 0.000000000000000000, 0.000000000000000000, 1.000000000000000000 ) ) ;
#12927=DIRECTION ( 'NONE',  ( 0.000000000000000000, 0.000000000000000000, -1.000000000000000000 ) ) ;
#13009=VERTEX_POINT ( 'NONE', #13180 ) ;
#13018=CARTESIAN_POINT ( 'NONE',  ( 21.09785597605720042, -13.37218737171702543, 102.7370144706720225 ) ) ;
#13036=CARTESIAN_POINT ( 'NONE',  ( 21.09785597605719332, 17.36451738380053555, 34.36516646732340519 ) ) ;
#13061=DIRECTION ( 'NONE',  ( 0.000000000000000000, 1.000000000000000000, -0.000000000000000000 ) ) ;
#13064=DIRECTION ( 'NONE',  ( -1.000000000000000000, 0.000000000000000000, 0.000000000000000000 ) ) ;
#13073=AXIS2_PLACEMENT_3D ( 'NONE', #5094, #20337, #17888 ) ;
#13075=AXIS2_PLACEMENT_3D ( 'NONE', #17403, #4116, #32022 ) ;
#13085=ORIENTED_EDGE ( 'NONE', *, *, #6937, .T. ) ;
#13108=ORIENTED_EDGE ( 'NONE', *, *, #22863, .T. ) ;
#13127=CARTESIAN_POINT ( 'NONE',  ( 21.09785597605720042, -13.88867167006704939, -11.65212399594570769 ) ) ;
#13150=STYLED_ITEM('',(#32522),#12396);
#13160=LINE ( 'NONE', #13327, #2768 ) ;
#13164=DIRECTION ( 'NONE',  ( 0.000000000000000000, 1.000000000000000000, -0.000000000000000000 ) ) ;
#13180=CARTESIAN_POINT ( 'NONE',  ( 21.09785597605720042, -13.59284023713420630, -8.574624342367267005 ) ) ;
#13190=ADVANCED_FACE ( 'NONE', ( #24299 ), #1496, .T. ) ;
#13208=EDGE_CURVE ( 'NONE', #14178, #24256, #16700, .T. ) ;
#13233=EDGE_LOOP ( 'NONE', ( #24121, #14514, #32128, #26651 ) ) ;
#13268=CIRCLE ( 'NONE', #8028, 58.66319174311612272 ) ;
#13274=AXIS2_PLACEMENT_3D ( 'NONE', #15882, #30818, #23425 ) ;
#13312=ORIENTED_EDGE ( 'NONE', *, *, #5037, .T. ) ;
#13321=EDGE_CURVE ( 'NONE', #8764, #20587, #17772, .T. ) ;
#13327=CARTESIAN_POINT ( 'NONE',  ( 21.09785597605720042, -13.98292989133646103, 105.7214871010043709 ) ) ;
#13338=CARTESIAN_POINT ( 'NONE',  ( 71.26428788917345969, -13.30632128221581212, 71.78284114260775084 ) ) ;
#13353=CARTESIAN_POINT ( 'NONE',  ( 21.09785597605718621, 7.237299147902269247, 66.50898490448155087 ) ) ;
#13421=DIRECTION ( 'NONE',  ( 0.000000000000000000, 0.000000000000000000, -1.000000000000000000 ) ) ;
#13476=CARTESIAN_POINT ( 'NONE',  ( 21.09785597605719332, 15.24673779880127178, 34.56516646732339382 ) ) ;
#13477=ORIENTED_EDGE ( 'NONE', *, *, #16806, .T. ) ;
#13505=CIRCLE ( 'NONE', #17682, 0.1999999999999987899 ) ;
#13518=CARTESIAN_POINT ( 'NONE',  ( 21.09785597605719332, -13.74048473023143835, -11.17459240385188934 ) ) ;
#13534=ORIENTED_EDGE ( 'NONE', *, *, #29693, .F. ) ;
#13539=EDGE_LOOP ( 'NONE', ( #4278, #19199, #9358, #25322 ) ) ;
#13568=DIRECTION ( 'NONE',  ( -1.102049569453931065E-16, 0.000000000000000000, 1.000000000000000000 ) ) ;
#13592=ORIENTED_EDGE ( 'NONE', *, *, #15628, .T. ) ;
#13635=CARTESIAN_POINT ( 'NONE',  ( -27.33830150920368496, -13.30632128221581212, 75.01995691340935934 ) ) ;
#13644=DIRECTION ( 'NONE',  ( -0.000000000000000000, -1.000000000000000000, -0.000000000000000000 ) ) ;
#13661=CARTESIAN_POINT ( 'NONE',  ( 21.09785597605719332, 7.094379510609982731, 47.04930799450051637 ) ) ;
#13674=EDGE_CURVE ( 'NONE', #26992, #12577, #28801, .T. ) ;
#13687=LINE ( 'NONE', #21202, #19466 ) ;
#13699=ORIENTED_EDGE ( 'NONE', *, *, #20082, .F. ) ;
#13705=FACE_OUTER_BOUND ( 'NONE', #29891, .T. ) ;
#13713=DIRECTION ( 'NONE',  ( 0.000000000000000000, 1.000000000000000000, -0.000000000000000000 ) ) ;
#13734=LINE ( 'NONE', #24216, #8979 ) ;
#13748=AXIS2_PLACEMENT_3D ( 'NONE', #4645, #9900, #5137 ) ;
#13755=AXIS2_PLACEMENT_3D ( 'NONE', #30201, #17554, #20177 ) ;
#13787=AXIS2_PLACEMENT_3D ( 'NONE', #3290, #18384, #675 ) ;
#13792=CARTESIAN_POINT ( 'NONE',  ( 21.09785597605719332, 6.547041198165487685, 26.66847926540309288 ) ) ;
#13795=CARTESIAN_POINT ( 'NONE',  ( 3.114080794088355475, -13.30632128221581389, 100.0115811999271500 ) ) ;
#13817=CARTESIAN_POINT ( 'NONE',  ( 36.19429842010744380, -13.74047052604243113, -9.312396943078796951 ) ) ;
#13820=ORIENTED_EDGE ( 'NONE', *, *, #13674, .T. ) ;
#13835=CARTESIAN_POINT ( 'NONE',  ( 21.09785597605719332, 15.43591091851532759, 47.04930799450051637 ) ) ;
#13896=DIRECTION ( 'NONE',  ( -0.000000000000000000, -1.000000000000000000, -0.000000000000000000 ) ) ;
#13906=AXIS2_PLACEMENT_3D ( 'NONE', #23327, #8553, #838 ) ;
#13910=VECTOR ( 'NONE', #12298, 1000.000000000000000 ) ;
#13919=FACE_OUTER_BOUND ( 'NONE', #14893, .T. ) ;
#13956=DIRECTION ( 'NONE',  ( 1.224646799147353207E-16, -0.000000000000000000, -1.000000000000000000 ) ) ;
#13969=CARTESIAN_POINT ( 'NONE',  ( 21.09785597605719332, 15.24673779880127356, 47.04930799450051637 ) ) ;
#13974=CARTESIAN_POINT ( 'NONE',  ( 55.14312657641617932, -13.30632128221581212, 2.672082950226034370 ) ) ;
#13982=CARTESIAN_POINT ( 'NONE',  ( 21.09785597605719332, 17.16451738380053627, 59.53344952167761761 ) ) ;
#14004=VERTEX_POINT ( 'NONE', #5144 ) ;
#14008=EDGE_CURVE ( 'NONE', #26439, #28177, #17837, .T. ) ;
#14024=AXIS2_PLACEMENT_3D ( 'NONE', #1046, #23693, #11072 ) ;
#14029=DIRECTION ( 'NONE',  ( -0.000000000000000000, -1.000000000000000000, -0.000000000000000000 ) ) ;
#14050=AXIS2_PLACEMENT_3D ( 'NONE', #16160, #11246, #28163 ) ;
#14065=UNCERTAINTY_MEASURE_WITH_UNIT (LENGTH_MEASURE( 1.000000000000000082E-05 ), #9888, 'distance_accuracy_value', 'NONE');
#14070=CIRCLE ( 'NONE', #24765, 1.000000000001013856 ) ;
#14077=DIRECTION ( 'NONE',  ( -1.096245967261387844E-16, 0.000000000000000000, 1.000000000000000000 ) ) ;
#14145=DIRECTION ( 'NONE',  ( 1.000000000000000000, 0.000000000000000000, -1.224646799147353207E-16 ) ) ;
#14166=EDGE_CURVE ( 'NONE', #32191, #13009, #24633, .T. ) ;
#14178=VERTEX_POINT ( 'NONE', #18534 ) ;
#14189=DIRECTION ( 'NONE',  ( 0.000000000000000000, -0.000000000000000000, -1.000000000000000000 ) ) ;
#14200=DIRECTION ( 'NONE',  ( 0.000000000000000000, 1.000000000000000000, -0.000000000000000000 ) ) ;
#14235=TOROIDAL_SURFACE ( 'NONE', #26292, 70.59901951359279337, 0.6000000000000020872 ) ;
#14245=VERTEX_POINT ( 'NONE', #13476 ) ;
#14247=ORIENTED_EDGE ( 'NONE', *, *, #8083, .T. ) ;
#14249=TOROIDAL_SURFACE ( 'NONE', #27345, 58.88977237527051756, 0.9999999999999997780 ) ;
#14296=CARTESIAN_POINT ( 'NONE',  ( 74.06012918148380209, -13.30632128221581212, 29.06553281253166432 ) ) ;
#14308=DIRECTION ( 'NONE',  ( 0.000000000000000000, 0.000000000000000000, -1.000000000000000000 ) ) ;
#14309=AXIS2_PLACEMENT_3D ( 'NONE', #7977, #17968, #10113 ) ;
#14314=CARTESIAN_POINT ( 'NONE',  ( 21.09785597605720042, -16.03545420775220265, -23.54971151909227700 ) ) ;
#14320=CIRCLE ( 'NONE', #32156, 12.48414152717711900 ) ;
#14328=AXIS2_PLACEMENT_3D ( 'NONE', #16059, #26064, #8684 ) ;
#14342=EDGE_LOOP ( 'NONE', ( #8710, #2241, #17183, #27147 ) ) ;
#14390=EDGE_CURVE ( 'NONE', #15932, #15162, #21496, .T. ) ;
#14426=CIRCLE ( 'NONE', #4988, 36.01080762834750715 ) ;
#14445=VERTEX_POINT ( 'NONE', #24599 ) ;
#14447=CARTESIAN_POINT ( 'NONE',  ( 21.09785597605718976, 7.094379510609982731, 66.36907787364950195 ) ) ;
#14461=CARTESIAN_POINT ( 'NONE',  ( 49.06850489496601142, -13.30632128221581034, -1.386849490760364789 ) ) ;
#14514=ORIENTED_EDGE ( 'NONE', *, *, #19061, .F. ) ;
#14537=CARTESIAN_POINT ( 'NONE',  ( 21.09785597605719332, 38.31023907818019580, 47.04930799450051637 ) ) ;
#14551=CONICAL_SURFACE ( 'NONE', #394, 19.45967690998103805, 0.7960495370845414032 ) ;
#14552=AXIS2_PLACEMENT_3D ( 'NONE', #24833, #21701, #1852 ) ;
#14554=ORIENTED_EDGE ( 'NONE', *, *, #31790, .F. ) ;
#14609=LINE ( 'NONE', #4431, #16992 ) ;
#14610=EDGE_LOOP ( 'NONE', ( #15893, #12217, #32246, #25062 ) ) ;
#14613=DIRECTION ( 'NONE',  ( 0.000000000000000000, -0.000000000000000000, -1.000000000000000000 ) ) ;
#14617=EDGE_CURVE ( 'NONE', #6215, #6567, #28711, .T. ) ;
#14619=ORIENTED_EDGE ( 'NONE', *, *, #28988, .T. ) ;
#14638=ADVANCED_FACE ( 'NONE', ( #3365 ), #20312, .F. ) ;
#14648=CIRCLE ( 'NONE', #32482, 0.2000000000000057288 ) ;
#14652=CARTESIAN_POINT ( 'NONE',  ( 6.001413532006936613, -13.74047052604243646, -9.312396943078789846 ) ) ;
#14703=CARTESIAN_POINT ( 'NONE',  ( 21.09785597605720042, -14.24176827912842391, -11.80059343253840609 ) ) ;
#14726=TOROIDAL_SURFACE ( 'NONE', #19959, 83.95481021798164534, 94.94530576803616384 ) ;
#14731=AXIS2_PLACEMENT_3D ( 'NONE', #4351, #6811, #16813 ) ;
#14748=CARTESIAN_POINT ( 'NONE',  ( 21.09785597605719332, 14.58544108513610027, 47.04930799450051637 ) ) ;
#14767=AXIS2_PLACEMENT_3D ( 'NONE', #12771, #17998, #608 ) ;
#14769=DIRECTION ( 'NONE',  ( 0.000000000000000000, -1.000000000000000000, 0.000000000000000000 ) ) ;
#14784=SHAPE_DEFINITION_REPRESENTATION ( #2233, #21423 ) ;
#14788=CARTESIAN_POINT ( 'NONE',  ( 21.09785597605720042, -16.63545420775220407, 47.04930799450051637 ) ) ;
#14815=CARTESIAN_POINT ( 'NONE',  ( -14.41812891119676188, -13.74047052604243646, 0.7550407962218198543 ) ) ;
#14820=AXIS2_PLACEMENT_3D ( 'NONE', #2330, #12347, #22340 ) ;
#14823=VERTEX_POINT ( 'NONE', #12552 ) ;
#14847=EDGE_CURVE ( 'NONE', #3864, #26992, #1456, .T. ) ;
#14858=DIRECTION ( 'NONE',  ( -0.000000000000000000, -1.000000000000000000, -0.000000000000000000 ) ) ;
#14863=DIRECTION ( 'NONE',  ( 0.000000000000000000, 0.000000000000000000, -1.000000000000000000 ) ) ;
#14867=VERTEX_POINT ( 'NONE', #13036 ) ;
#14893=EDGE_LOOP ( 'NONE', ( #3453, #21649, #27667, #3028 ) ) ;
#14896=DIRECTION ( 'NONE',  ( 0.000000000000000000, 0.000000000000000000, -1.000000000000000000 ) ) ;
#14928=DIRECTION ( 'NONE',  ( -0.000000000000000000, -1.000000000000000000, -0.000000000000000000 ) ) ;
#14944=VERTEX_POINT ( 'NONE', #3813 ) ;
#14969=DIRECTION ( 'NONE',  ( 0.000000000000000000, 0.000000000000000000, 1.000000000000000000 ) ) ;
#14976=CARTESIAN_POINT ( 'NONE',  ( 21.09785597605720042, -14.04221034894631615, -11.61388374861560635 ) ) ;
#14998=EDGE_CURVE ( 'NONE', #4372, #11143, #7252, .T. ) ;
#14999=CARTESIAN_POINT ( 'NONE',  ( 21.09785597605720753, -16.03545420775220265, 117.0483275080932941 ) ) ;
#15001=AXIS2_PLACEMENT_3D ( 'NONE', #1219, #13713, #10776 ) ;
#15064=CARTESIAN_POINT ( 'NONE',  ( 21.09785597605720042, -13.40182760052194588, -8.733904799977112887 ) ) ;
#15071=CARTESIAN_POINT ( 'NONE',  ( 21.09785597605719332, 15.43591091851533115, 47.04930799450051637 ) ) ;
#15073=DIRECTION ( 'NONE',  ( -0.000000000000000000, -1.000000000000000000, -0.000000000000000000 ) ) ;
#15102=ORIENTED_EDGE ( 'NONE', *, *, #10321, .F. ) ;
#15113=CARTESIAN_POINT ( 'NONE',  ( 21.09785597605719332, 6.574714862014670480, 47.04930799450051637 ) ) ;
#15154=FACE_OUTER_BOUND ( 'NONE', #30944, .T. ) ;
#15162=VERTEX_POINT ( 'NONE', #6761 ) ;
#15168=EDGE_CURVE ( 'NONE', #32483, #22659, #2542, .T. ) ;
#15218=FACE_OUTER_BOUND ( 'NONE', #415, .T. ) ;
#15229=CIRCLE ( 'NONE', #17320, 94.44530576803552435 ) ;
#15263=EDGE_CURVE ( 'NONE', #22659, #7408, #28228, .T. ) ;
#15275=CIRCLE ( 'NONE', #26276, 0.1999999999999987899 ) ;
#15298=DIRECTION ( 'NONE',  ( 0.000000000000000000, 0.000000000000000000, 1.000000000000000000 ) ) ;
#15302=SHAPE_REPRESENTATION_RELATIONSHIP ( 'NONE' , 'NONE' ,  #21423, #8462 ) ;
#15318=EDGE_CURVE ( 'NONE', #27142, #30184, #14070, .T. ) ;
#15330=B_SPLINE_CURVE_WITH_KNOTS ( 'NONE', 3,
 ( #31722, #9235, #19063, #19223, #29248, #19395, #29586, #31563, #7093, #6931, #4797, #26951, #24322, #29747, #6767, #22015, #27113, #27277, #9396, #16768, #29092, #31879, #7262, #6610, #21527, #19720, #14815, #32047, #9562, #19557, #14652, #16602, #26623, #1842 ),
 .UNSPECIFIED., .F., .F.,
 ( 4, 2, 2, 2, 2, 2, 2, 2, 2, 2, 2, 2, 2, 2, 2, 2, 4 ),
 ( 0.5000000000000000000, 0.5312500000000000000, 0.5625000000000000000, 0.5937500000000000000, 0.6250000000000000000, 0.6562500000000000000, 0.6875000000000000000, 0.7187500000000000000, 0.7500000000000000000, 0.7812500000000000000, 0.8125000000000000000, 0.8437500000000000000, 0.8750000000000000000, 0.9062500000000000000, 0.9375000000000000000, 0.9687500000000000000, 1.000000000000000000 ),
 .UNSPECIFIED. ) ;
#15351=ADVANCED_FACE ( 'NONE', ( #7255 ), #22683, .T. ) ;
#15355=AXIS2_PLACEMENT_3D ( 'NONE', #17708, #27733, #806 ) ;
#15383=CARTESIAN_POINT ( 'NONE',  ( 21.09785597605718621, 77.37241625295546044, 47.04930799450051637 ) ) ;
#15400=EDGE_CURVE ( 'NONE', #7489, #15932, #13160, .T. ) ;
#15411=ADVANCED_FACE ( 'NONE', ( #11016, #30718 ), #25463, .T. ) ;
#15416=VERTEX_POINT ( 'NONE', #21004 ) ;
#15450=EDGE_CURVE ( 'NONE', #11333, #20809, #24239, .T. ) ;
#15459=PRESENTATION_STYLE_ASSIGNMENT (( #29923 ) ) ;
#15472=AXIS2_PLACEMENT_3D ( 'NONE', #25942, #13164, #10540 ) ;
#15573=DIRECTION ( 'NONE',  ( 0.000000000000000000, 0.000000000000000000, -1.000000000000000000 ) ) ;
#15585=VERTEX_POINT ( 'NONE', #32491 ) ;
#15592=AXIS2_PLACEMENT_3D ( 'NONE', #851, #10876, #20867 ) ;
#15628=EDGE_CURVE ( 'NONE', #25082, #9462, #13268, .T. ) ;
#15631=EDGE_CURVE ( 'NONE', #27949, #29666, #22129, .T. ) ;
#15670=EDGE_LOOP ( 'NONE', ( #20837, #12376, #7121, #18030 ) ) ;
#15673=CONICAL_SURFACE ( 'NONE', #1506, 19.45967690998103805, 0.7960495370845414032 ) ;
#15751=CARTESIAN_POINT ( 'NONE',  ( 21.09785597605720042, -13.59284023713420630, 47.04930799450051637 ) ) ;
#15762=CIRCLE ( 'NONE', #13075, 12.48414152717711190 ) ;
#15775=DIRECTION ( 'NONE',  ( 0.000000000000000000, 1.000000000000000000, 0.000000000000000000 ) ) ;
#15776=CARTESIAN_POINT ( 'NONE',  ( 21.09785597605718621, 77.37241625295546044, 47.04930799450051637 ) ) ;
#15802=EDGE_CURVE ( 'NONE', #13009, #32191, #3843, .T. ) ;
#15805=AXIS2_PLACEMENT_3D ( 'NONE', #4852, #88, #27501 ) ;
#15826=DIRECTION ( 'NONE',  ( 0.000000000000000000, 1.000000000000000000, -0.000000000000000000 ) ) ;
#15853=EDGE_CURVE ( 'NONE', #22659, #32483, #2247, .T. ) ;
#15858=FACE_OUTER_BOUND ( 'NONE', #31411, .T. ) ;
#15869=DIRECTION ( 'NONE',  ( 0.000000000000000000, 0.000000000000000000, -1.000000000000000000 ) ) ;
#15872=EDGE_CURVE ( 'NONE', #27142, #14245, #14320, .T. ) ;
#15874=( NAMED_UNIT ( * ) PLANE_ANGLE_UNIT ( ) SI_UNIT ( $, .RADIAN. ) );
#15880=LINE ( 'NONE', #16658, #27707 ) ;
#15882=CARTESIAN_POINT ( 'NONE',  ( 21.09785597605720753, -16.03545420775220265, 117.6483275080933169 ) ) ;
#15893=ORIENTED_EDGE ( 'NONE', *, *, #23902, .F. ) ;
#15895=AXIS2_PLACEMENT_3D ( 'NONE', #21716, #1531, #19416 ) ;
#15897=FACE_OUTER_BOUND ( 'NONE', #3197, .T. ) ;
#15914=ORIENTED_EDGE ( 'NONE', *, *, #21807, .T. ) ;
#15926=CARTESIAN_POINT ( 'NONE',  ( 21.09785597605719687, -13.30631372918550959, 102.8621366805641770 ) ) ;
#15927=CARTESIAN_POINT ( 'NONE',  ( 21.09785597605718976, 6.574714862014670480, 26.91277942630439668 ) ) ;
#15931=ADVANCED_FACE ( 'NONE', ( #13919 ), #19549, .T. ) ;
#15932=VERTEX_POINT ( 'NONE', #8984 ) ;
#15944=CARTESIAN_POINT ( 'NONE',  ( 21.09785597605720042, -13.40182760052194588, 47.04930799450051637 ) ) ;
#15955=TOROIDAL_SURFACE ( 'NONE', #7058, 58.03288776117695846, 0.1999999999999970968 ) ;
#15977=CARTESIAN_POINT ( 'NONE',  ( 21.09785597605720042, -13.98292989133646103, 47.04930799450051637 ) ) ;
#15980=AXIS2_PLACEMENT_3D ( 'NONE', #20781, #28652, #12927 ) ;
#16012=CARTESIAN_POINT ( 'NONE',  ( 21.09785597605720042, -13.64309448858209528, 47.04930799450051637 ) ) ;
#16019=FACE_OUTER_BOUND ( 'NONE', #11992, .T. ) ;
#16052=ORIENTED_EDGE ( 'NONE', *, *, #6004, .T. ) ;
#16059=CARTESIAN_POINT ( 'NONE',  ( 21.09785597605719332, 14.77310068074637961, 47.04930799450051637 ) ) ;
#16146=ORIENTED_EDGE ( 'NONE', *, *, #10409, .T. ) ;
#16150=ADVANCED_FACE ( 'NONE', ( #22911 ), #24225, .F. ) ;
#16160=CARTESIAN_POINT ( 'NONE',  ( 21.09785597605720042, -13.68834655544033652, 47.04930799450051637 ) ) ;
#16212=CARTESIAN_POINT ( 'NONE',  ( 21.09785597605718621, 77.37241625295546044, -36.90555089683208223 ) ) ;
#16239=AXIS2_PLACEMENT_3D ( 'NONE', #18919, #26324, #9086 ) ;
#16243=CARTESIAN_POINT ( 'NONE',  ( 3.114080794088308846, -13.30632128221581034, -5.912965210926084403 ) ) ;
#16282=FACE_OUTER_BOUND ( 'NONE', #23170, .T. ) ;
#16292=CARTESIAN_POINT ( 'NONE',  ( 21.09785597605720753, -13.64309448858209528, 105.9390803697710339 ) ) ;
#16353=TOROIDAL_SURFACE ( 'NONE', #27918, 78.39999999999999147, 0.1000000000000014211 ) ;
#16369=CARTESIAN_POINT ( 'NONE',  ( 21.09785597605719332, 7.264443105416139801, 47.04930799450051637 ) ) ;
#16404=CARTESIAN_POINT ( 'NONE',  ( -31.86441722936942611, -13.30632128221581212, 29.06553281253165011 ) ) ;
#16405=DIRECTION ( 'NONE',  ( 0.000000000000000000, 1.000000000000000000, -0.000000000000000000 ) ) ;
#16410=FACE_OUTER_BOUND ( 'NONE', #4865, .T. ) ;
#16418=CARTESIAN_POINT ( 'NONE',  ( 57.98048228007293403, -13.30632128221581034, 5.000640598253887070 ) ) ;
#16431=DIRECTION ( 'NONE',  ( 1.000000000000000000, 0.000000000000000000, -1.224646799147353207E-16 ) ) ;
#16457=FACE_OUTER_BOUND ( 'NONE', #24931, .T. ) ;
#16467=DIRECTION ( 'NONE',  ( 1.000000000000000000, 0.000000000000000000, 0.000000000000000000 ) ) ;
#16480=TOROIDAL_SURFACE ( 'NONE', #258, 83.95481021798164534, 94.94530576803560962 ) ;
#16502=CARTESIAN_POINT ( 'NONE',  ( 21.09785597605720042, -13.40182760052194588, 47.04930799450051637 ) ) ;
#16522=DIRECTION ( 'NONE',  ( -1.000000000000000000, 0.000000000000000000, -1.224646799147353207E-16 ) ) ;
#16553=ADVANCED_FACE ( 'NONE', ( #17061 ), #8006, .T. ) ;
#16568=DIRECTION ( 'NONE',  ( 0.000000000000000000, 0.000000000000000000, 1.000000000000000000 ) ) ;
#16569=DIRECTION ( 'NONE',  ( 0.000000000000000000, 0.000000000000000000, -1.000000000000000000 ) ) ;
#16574=CARTESIAN_POINT ( 'NONE',  ( 71.26428788917343127, -13.30632128221581212, 22.31577484639327125 ) ) ;
#16581=CARTESIAN_POINT ( 'NONE',  ( 77.45956091363649421, -13.74047052604243113, 62.14575043855074910 ) ) ;
#16592=CARTESIAN_POINT ( 'NONE',  ( 21.09785597605718976, -13.68121847681060643, 47.04930799450051637 ) ) ;
#16602=CARTESIAN_POINT ( 'NONE',  ( 13.47645946438857401, -13.74047052604243646, -10.79927602576051093 ) ) ;
#16618=CARTESIAN_POINT ( 'NONE',  ( 21.09785597605719332, 15.24673779880127178, 59.53344952167763182 ) ) ;
#16620=ADVANCED_FACE ( 'NONE', ( #4435 ), #27915, .T. ) ;
#16628=CIRCLE ( 'NONE', #14024, 78.50000000000000000 ) ;
#16632=DIRECTION ( 'NONE',  ( 0.000000000000000000, 0.000000000000000000, -1.000000000000000000 ) ) ;
#16643=FACE_OUTER_BOUND ( 'NONE', #4054, .T. ) ;
#16649=DIRECTION ( 'NONE',  ( -0.000000000000000000, -1.000000000000000000, -0.000000000000000000 ) ) ;
#16658=CARTESIAN_POINT ( 'NONE',  ( 21.09785597605719332, 34.11266481626051217, 34.06511779397349216 ) ) ;
#16663=VERTEX_POINT ( 'NONE', #26755 ) ;
#16700=CIRCLE ( 'NONE', #25106, 70.59901951359279337 ) ;
#16711=VERTEX_POINT ( 'NONE', #9848 ) ;
#16728=ORIENTED_EDGE ( 'NONE', *, *, #11928, .T. ) ;
#16733=EDGE_CURVE ( 'NONE', #24243, #30037, #10114, .T. ) ;
#16740=CARTESIAN_POINT ( 'NONE',  ( 76.34803497562474206, -13.74047052604243646, 65.80996039395137132 ) ) ;
#16757=AXIS2_PLACEMENT_3D ( 'NONE', #10743, #23365, #5485 ) ;
#16768=CARTESIAN_POINT ( 'NONE',  ( -35.26384896152210757, -13.74047052604243646, 31.95286555045027299 ) ) ;
#16775=TOROIDAL_SURFACE ( 'NONE', #3686, 19.31976987914897848, 0.2000000000000029809 ) ;
#16802=EDGE_CURVE ( 'NONE', #29052, #31613, #25842, .T. ) ;
#16806=EDGE_CURVE ( 'NONE', #14245, #27142, #24272, .T. ) ;
#16813=DIRECTION ( 'NONE',  ( 0.000000000000000000, 0.000000000000000000, -1.000000000000000000 ) ) ;
#16814=FACE_OUTER_BOUND ( 'NONE', #15670, .T. ) ;
#16820=CARTESIAN_POINT ( 'NONE',  ( 21.09785597605720042, -16.03545420775220265, -22.94971151909227203 ) ) ;
#16852=ORIENTED_EDGE ( 'NONE', *, *, #1399, .T. ) ;
#16853=CARTESIAN_POINT ( 'NONE',  ( 21.09785597605718266, -13.68121847681060643, 105.0821957556774890 ) ) ;
#16888=AXIS2_PLACEMENT_3D ( 'NONE', #12310, #32335, #7707 ) ;
#16919=DIRECTION ( 'NONE',  ( 0.000000000000000000, 1.000000000000000000, -0.000000000000000000 ) ) ;
#16946=EDGE_LOOP ( 'NONE', ( #27781, #19227, #2398, #21502 ) ) ;
#16976=DIRECTION ( 'NONE',  ( 0.000000000000000000, 1.000000000000000000, -0.000000000000000000 ) ) ;
#16979=ORIENTED_EDGE ( 'NONE', *, *, #30990, .F. ) ;
#16992=VECTOR ( 'NONE', #6727, 1000.000000000000000 ) ;
#16996=AXIS2_PLACEMENT_3D ( 'NONE', #27099, #31868, #11690 ) ;
#16998=ADVANCED_FACE ( 'NONE', ( #24250, #26554 ), #31488, .T. ) ;
#17015=CARTESIAN_POINT ( 'NONE',  ( 21.09785597605719332, 6.547041198165487685, 47.04930799450051637 ) ) ;
#17017=CIRCLE ( 'NONE', #1271, 19.25826962553310295 ) ;
#17028=CIRCLE ( 'NONE', #2884, 58.09216821878681003 ) ;
#17040=APPLICATION_CONTEXT ( 'automotive_design' ) ;
#17047=TOROIDAL_SURFACE ( 'NONE', #20717, 70.59901951359279337, 1.000000000000000444 ) ;
#17050=EDGE_LOOP ( 'NONE', ( #23950, #17198, #8403, #27248 ) ) ;
#17057=ORIENTED_EDGE ( 'NONE', *, *, #226, .F. ) ;
#17061=FACE_OUTER_BOUND ( 'NONE', #25788, .T. ) ;
#17085=CARTESIAN_POINT ( 'NONE',  ( 21.09785597605719687, -13.30631372918550959, 102.8621366805641770 ) ) ;
#17120=AXIS2_PLACEMENT_3D ( 'NONE', #31494, #11308, #26238 ) ;
#17139=CARTESIAN_POINT ( 'NONE',  ( 21.09785597605719332, 15.43591091851532759, 47.04930799450051637 ) ) ;
#17146=EDGE_CURVE ( 'NONE', #32483, #6923, #4873, .T. ) ;
#17151=EDGE_CURVE ( 'NONE', #20020, #20587, #4906, .T. ) ;
#17160=ORIENTED_EDGE ( 'NONE', *, *, #9028, .T. ) ;
#17176=DIRECTION ( 'NONE',  ( -0.000000000000000000, -1.000000000000000000, -0.000000000000000000 ) ) ;
#17183=ORIENTED_EDGE ( 'NONE', *, *, #13321, .T. ) ;
#17198=ORIENTED_EDGE ( 'NONE', *, *, #16806, .F. ) ;
#17204=CIRCLE ( 'NONE', #21389, 55.69429210806286079 ) ;
#17232=CARTESIAN_POINT ( 'NONE',  ( 24.90860134598590037, -13.74047052604243824, 105.2732083934160983 ) ) ;
#17287=DIRECTION ( 'NONE',  ( 0.000000000000000000, 1.000000000000000000, -0.000000000000000000 ) ) ;
#17320=AXIS2_PLACEMENT_3D ( 'NONE', #3544, #21097, #13568 ) ;
#17326=AXIS2_PLACEMENT_3D ( 'NONE', #11904, #2222, #22391 ) ;
#17330=ADVANCED_FACE ( 'NONE', ( #10948 ), #30070, .T. ) ;
#17335=FACE_OUTER_BOUND ( 'NONE', #10693, .T. ) ;
#17373=ORIENTED_EDGE ( 'NONE', *, *, #31790, .T. ) ;
#17377=ADVANCED_FACE ( 'NONE', ( #31135 ), #23241, .T. ) ;
#17378=DIRECTION ( 'NONE',  ( -1.000000000000000000, 0.000000000000000000, -1.224646799147353207E-16 ) ) ;
#17379=DIRECTION ( 'NONE',  ( 0.000000000000000000, 0.000000000000000000, -1.000000000000000000 ) ) ;
#17385=EDGE_LOOP ( 'NONE', ( #18698, #5103, #20975, #23061 ) ) ;
#17402=ORIENTED_EDGE ( 'NONE', *, *, #10231, .T. ) ;
#17403=CARTESIAN_POINT ( 'NONE',  ( 21.09785597605719332, 17.16451738380053627, 47.04930799450051637 ) ) ;
#17415=CARTESIAN_POINT ( 'NONE',  ( 21.09785597605720753, -13.98292989133646103, 105.7214871010043709 ) ) ;
#17418=DIRECTION ( 'NONE',  ( -1.000000000000000000, 0.000000000000000000, -1.224646799147353207E-16 ) ) ;
#17428=AXIS2_PLACEMENT_3D ( 'NONE', #7049, #24940, #27562 ) ;
#17430=( LENGTH_UNIT ( ) NAMED_UNIT ( * ) SI_UNIT ( .MILLI., .METRE. ) );
#17441=DIRECTION ( 'NONE',  ( -0.000000000000000000, -1.000000000000000000, -0.000000000000000000 ) ) ;
#17492=AXIS2_PLACEMENT_3D ( 'NONE', #4121, #16431, #19373 ) ;
#17497=EDGE_LOOP ( 'NONE', ( #8049, #29611, #20387, #22812 ) ) ;
#17506=DIRECTION ( 'NONE',  ( 0.000000000000000000, 1.000000000000000000, -0.000000000000000000 ) ) ;
#17543=CARTESIAN_POINT ( 'NONE',  ( 21.09785597605720042, -14.04221034894631615, 47.04930799450051637 ) ) ;
#17551=CIRCLE ( 'NONE', #10752, 20.13652856819611969 ) ;
#17554=DIRECTION ( 'NONE',  ( 1.000000000000000000, 0.000000000000000000, -1.224646799147353207E-16 ) ) ;
#17566=CARTESIAN_POINT ( 'NONE',  ( 21.09785597605720042, -13.68834655544033652, 47.04930799450051637 ) ) ;
#17591=( NAMED_UNIT ( * ) SI_UNIT ( $, .STERADIAN. ) SOLID_ANGLE_UNIT ( ) );
#17607=VERTEX_POINT ( 'NONE', #13353 ) ;
#17621=EDGE_CURVE ( 'NONE', #27142, #27524, #3645, .T. ) ;
#17648=ORIENTED_EDGE ( 'NONE', *, *, #20844, .T. ) ;
#17672=CARTESIAN_POINT ( 'NONE',  ( 21.09785597605720042, -14.54791319078308653, 47.04930799450051637 ) ) ;
#17682=AXIS2_PLACEMENT_3D ( 'NONE', #994, #25939, #3454 ) ;
#17708=CARTESIAN_POINT ( 'NONE',  ( 21.09785597605720042, -13.64309448858209528, -11.84046438077000118 ) ) ;
#17737=ORIENTED_EDGE ( 'NONE', *, *, #24979, .F. ) ;
#17739=CARTESIAN_POINT ( 'NONE',  ( 21.09785597605719332, 7.881678200673685630, 47.04930799450051637 ) ) ;
#17749=EDGE_CURVE ( 'NONE', #6225, #11078, #8146, .T. ) ;
#17760=CIRCLE ( 'NONE', #3077, 55.69429210806286079 ) ;
#17772=CIRCLE ( 'NONE', #1017, 0.1999999999999987899 ) ;
#17781=DIRECTION ( 'NONE',  ( -0.000000000000000000, -1.000000000000000000, -0.000000000000000000 ) ) ;
#17792=EDGE_CURVE ( 'NONE', #32191, #11333, #19128, .T. ) ;
#17837=CIRCLE ( 'NONE', #22538, 78.50000000000000000 ) ;
#17861=AXIS2_PLACEMENT_3D ( 'NONE', #17139, #16976, #9934 ) ;
#17876=ORIENTED_EDGE ( 'NONE', *, *, #31517, .T. ) ;
#17888=DIRECTION ( 'NONE',  ( 0.000000000000000000, 0.000000000000000000, -1.000000000000000000 ) ) ;
#17899=VECTOR ( 'NONE', #2203, 999.9999999999998863 ) ;
#17936=CARTESIAN_POINT ( 'NONE',  ( 21.09785597605720042, -16.93545420775220478, -31.35069200549948221 ) ) ;
#17942=DIRECTION ( 'NONE',  ( 0.000000000000000000, 1.000000000000000000, -0.000000000000000000 ) ) ;
#17953=DIRECTION ( 'NONE',  ( 0.000000000000000000, 0.000000000000000000, 1.000000000000000000 ) ) ;
#17968=DIRECTION ( 'NONE',  ( 0.000000000000000000, 1.000000000000000000, -0.000000000000000000 ) ) ;
#17985=ORIENTED_EDGE ( 'NONE', *, *, #3999, .F. ) ;
#17998=DIRECTION ( 'NONE',  ( 0.000000000000000000, 1.000000000000000000, -0.000000000000000000 ) ) ;
#18012=CARTESIAN_POINT ( 'NONE',  ( 21.09785597605720042, -16.73545420775220194, 47.04930799450051637 ) ) ;
#18020=ORIENTED_EDGE ( 'NONE', *, *, #6523, .T. ) ;
#18030=ORIENTED_EDGE ( 'NONE', *, *, #15450, .F. ) ;
#18054=VERTEX_POINT ( 'NONE', #13518 ) ;
#18083=ORIENTED_EDGE ( 'NONE', *, *, #3109, .F. ) ;
#18103=AXIS2_PLACEMENT_3D ( 'NONE', #20328, #8201, #31007 ) ;
#18106=ORIENTED_EDGE ( 'NONE', *, *, #18853, .T. ) ;
#18108=AXIS2_PLACEMENT_3D ( 'NONE', #26505, #1547, #21566 ) ;
#18112=FACE_BOUND ( 'NONE', #18453, .T. ) ;
#18132=DIRECTION ( 'NONE',  ( 0.000000000000000000, 0.000000000000000000, -1.000000000000000000 ) ) ;
#18140=DIRECTION ( 'NONE',  ( -0.000000000000000000, -1.000000000000000000, -0.000000000000000000 ) ) ;
#18146=ORIENTED_EDGE ( 'NONE', *, *, #3822, .F. ) ;
#18283=ORIENTED_EDGE ( 'NONE', *, *, #15631, .T. ) ;
#18294=AXIS2_PLACEMENT_3D ( 'NONE', #29401, #19203, #29230 ) ;
#18311=ORIENTED_EDGE ( 'NONE', *, *, #18853, .F. ) ;
#18358=DIRECTION ( 'NONE',  ( 0.000000000000000000, 0.000000000000000000, -1.000000000000000000 ) ) ;
#18375=VERTEX_POINT ( 'NONE', #506 ) ;
#18377=CARTESIAN_POINT ( 'NONE',  ( 21.09785597605720042, -13.68834655544033652, -8.644984113562347972 ) ) ;
#18384=DIRECTION ( 'NONE',  ( 0.000000000000000000, -1.000000000000000000, -0.000000000000000000 ) ) ;
#18397=CARTESIAN_POINT ( 'NONE',  ( 65.47508102033168598, -13.30632128221581212, 81.09457859485948461 ) ) ;
#18413=VECTOR ( 'NONE', #13896, 1000.000000000000000 ) ;
#18439=CIRCLE ( 'NONE', #13748, 0.1999999999999987899 ) ;
#18447=EDGE_CURVE ( 'NONE', #14944, #31146, #3915, .T. ) ;
#18450=ADVANCED_FACE ( 'NONE', ( #20362 ), #8120, .F. ) ;
#18453=EDGE_LOOP ( 'NONE', ( #8453, #30088 ) ) ;
#18461=DIRECTION ( 'NONE',  ( 1.000000000000000000, 0.000000000000000000, 1.900504084856170908E-16 ) ) ;
#18477=EDGE_CURVE ( 'NONE', #23177, #6352, #29605, .T. ) ;
#18498=AXIS2_PLACEMENT_3D ( 'NONE', #1427, #26219, #3735 ) ;
#18530=CIRCLE ( 'NONE', #7007, 0.1999999999999918510 ) ;
#18534=CARTESIAN_POINT ( 'NONE',  ( 21.09785597605720042, -16.63545420775220407, -23.54971151909227700 ) ) ;
#18535=EDGE_LOOP ( 'NONE', ( #30189, #24281, #12796, #2140 ) ) ;
#18536=CARTESIAN_POINT ( 'NONE',  ( 17.44491328785236561, -13.30632128221581212, -8.763545028782028012 ) ) ;
#18538=DIRECTION ( 'NONE',  ( -0.000000000000000000, -1.000000000000000000, -0.000000000000000000 ) ) ;
#18605=ORIENTED_EDGE ( 'NONE', *, *, #25304, .T. ) ;
#18606=VERTEX_POINT ( 'NONE', #1916 ) ;
#18609=AXIS2_PLACEMENT_3D ( 'NONE', #9847, #32174, #25108 ) ;
#18618=EDGE_CURVE ( 'NONE', #16711, #7489, #22796, .T. ) ;
#18634=DIRECTION ( 'NONE',  ( 1.169615070119504008E-16, -0.2964022880492265255, 0.9550631830613005580 ) ) ;
#18646=PRODUCT_DEFINITION_CONTEXT ( 'detailed design', #23750, 'design' ) ;
#18655=( GEOMETRIC_REPRESENTATION_CONTEXT ( 3 ) GLOBAL_UNCERTAINTY_ASSIGNED_CONTEXT ( ( #21595 ) ) GLOBAL_UNIT_ASSIGNED_CONTEXT ( ( #17430, #27453, #17591 ) ) REPRESENTATION_CONTEXT ( 'NONE', 'WORKASPACE' ) );
#18661=CARTESIAN_POINT ( 'NONE',  ( 21.09785597605720042, -13.59284023713420630, 47.04930799450051637 ) ) ;
#18671=DIRECTION ( 'NONE',  ( 0.000000000000000000, 1.000000000000000000, -0.000000000000000000 ) ) ;
#18688=EDGE_LOOP ( 'NONE', ( #21587, #12787, #22489, #28535 ) ) ;
#18698=ORIENTED_EDGE ( 'NONE', *, *, #4545, .T. ) ;
#18738=DIRECTION ( 'NONE',  ( -8.751303817264967506E-17, -0.6995351541602693457, -0.7145981864614324719 ) ) ;
#18742=AXIS2_PLACEMENT_3D ( 'NONE', #29724, #22479, #170 ) ;
#18760=CARTESIAN_POINT ( 'NONE',  ( 21.09785597605718976, -13.68121847681060643, 47.04930799450051637 ) ) ;
#18802=ADVANCED_FACE ( 'NONE', ( #3536 ), #17047, .T. ) ;
#18818=ORIENTED_EDGE ( 'NONE', *, *, #5908, .T. ) ;
#18841=FACE_OUTER_BOUND ( 'NONE', #23596, .T. ) ;
#18850=EDGE_LOOP ( 'NONE', ( #10463, #9982, #8533, #31708 ) ) ;
#18853=EDGE_CURVE ( 'NONE', #23707, #9682, #27544, .T. ) ;
#18858=CARTESIAN_POINT ( 'NONE',  ( -20.95081142018943510, -13.30632128221581212, 10.16668169048477566 ) ) ;
#18866=DIRECTION ( 'NONE',  ( 0.000000000000000000, 1.000000000000000000, -0.000000000000000000 ) ) ;
#18873=AXIS2_PLACEMENT_3D ( 'NONE', #26417, #21314, #31350 ) ;
#18883=TOROIDAL_SURFACE ( 'NONE', #18294, 64.50000000000000000, 5.099019513592785380 ) ;
#18902=AXIS2_PLACEMENT_3D ( 'NONE', #12740, #85, #10107 ) ;
#18918=ORIENTED_EDGE ( 'NONE', *, *, #15872, .T. ) ;
#18919=CARTESIAN_POINT ( 'NONE',  ( 21.09785597605719332, 6.547041198165487685, 47.04930799450051637 ) ) ;
#18930=ORIENTED_EDGE ( 'NONE', *, *, #10954, .F. ) ;
#18981=ORIENTED_EDGE ( 'NONE', *, *, #12621, .F. ) ;
#19022=ADVANCED_FACE ( 'NONE', ( #32420 ), #23843, .T. ) ;
#19027=DIRECTION ( 'NONE',  ( -1.000000000000000000, 0.000000000000000000, 0.000000000000000000 ) ) ;
#19040=DIRECTION ( 'NONE',  ( 0.000000000000000000, 0.000000000000000000, 1.000000000000000000 ) ) ;
#19061=EDGE_CURVE ( 'NONE', #7489, #16711, #11297, .T. ) ;
#19063=CARTESIAN_POINT ( 'NONE',  ( 13.47645946438859355, -13.74047052604243646, 104.8978920147615810 ) ) ;
#19064=DIRECTION ( 'NONE',  ( 0.000000000000000000, 1.000000000000000000, -0.000000000000000000 ) ) ;
#19085=ORIENTED_EDGE ( 'NONE', *, *, #32211, .T. ) ;
#19092=CARTESIAN_POINT ( 'NONE',  ( 21.09785597605719332, 34.11266481626051217, 47.04930799450051637 ) ) ;
#19094=CIRCLE ( 'NONE', #13906, 70.59901951359279337 ) ;
#19106=DIRECTION ( 'NONE',  ( -0.000000000000000000, -1.000000000000000000, -0.000000000000000000 ) ) ;
#19128=CIRCLE ( 'NONE', #18108, 0.1000000000000028644 ) ;
#19174=STYLED_ITEM ( 'NONE', ( #15459 ), #8462 ) ;
#19199=ORIENTED_EDGE ( 'NONE', *, *, #23938, .F. ) ;
#19201=CARTESIAN_POINT ( 'NONE',  ( 56.61384086331115384, -13.74047052604243646, 0.7550407962218190772 ) ) ;
#19203=DIRECTION ( 'NONE',  ( -0.000000000000000000, -1.000000000000000000, -0.000000000000000000 ) ) ;
#19223=CARTESIAN_POINT ( 'NONE',  ( 6.001413532006956153, -13.74047052604243468, 103.4110129320797853 ) ) ;
#19227=ORIENTED_EDGE ( 'NONE', *, *, #17621, .T. ) ;
#19289=UNCERTAINTY_MEASURE_WITH_UNIT (LENGTH_MEASURE( 1.000000000000000082E-05 ), #28350, 'distance_accuracy_value', 'NONE');
#19339=TOROIDAL_SURFACE ( 'NONE', #8338, 58.03288776117695846, 0.1999999999999970968 ) ;
#19356=DIRECTION ( 'NONE',  ( 1.000000000000000000, 0.000000000000000000, 0.000000000000000000 ) ) ;
#19364=CARTESIAN_POINT ( 'NONE',  ( 21.09785597605720042, -16.93545420775220478, 47.04930799450051637 ) ) ;
#19369=DIRECTION ( 'NONE',  ( 0.000000000000000000, 0.000000000000000000, -1.000000000000000000 ) ) ;
#19373=DIRECTION ( 'NONE',  ( 0.000000000000000000, 0.000000000000000000, -1.000000000000000000 ) ) ;
#19395=CARTESIAN_POINT ( 'NONE',  ( -4.704135725172196025, -13.74047052604243646, 99.38286875800066866 ) ) ;
#19416=DIRECTION ( 'NONE',  ( 0.000000000000000000, 0.000000000000000000, -1.000000000000000000 ) ) ;
#19449=( NAMED_UNIT ( * ) SI_UNIT ( $, .STERADIAN. ) SOLID_ANGLE_UNIT ( ) );
#19455=CIRCLE ( 'NONE', #30483, 1.000000000000000888 ) ;
#19460=ORIENTED_EDGE ( 'NONE', *, *, #9426, .T. ) ;
#19466=VECTOR ( 'NONE', #18738, 1000.000000000000114 ) ;
#19527=ORIENTED_EDGE ( 'NONE', *, *, #21962, .F. ) ;
#19546=ORIENTED_EDGE ( 'NONE', *, *, #12628, .F. ) ;
#19549=TOROIDAL_SURFACE ( 'NONE', #30569, 58.88977237527051756, 0.9999999999999997780 ) ;
#19557=CARTESIAN_POINT ( 'NONE',  ( 2.337203576606295297, -13.74047052604243646, -8.200871005066998620 ) ) ;
#19559=EDGE_CURVE ( 'NONE', #7408, #6923, #3408, .T. ) ;
#19588=AXIS2_PLACEMENT_3D ( 'NONE', #27749, #4781, #29897 ) ;
#19606=CARTESIAN_POINT ( 'NONE',  ( 21.09785597605719332, -12.82881809906321458, 47.04930799450051637 ) ) ;
#19607=ORIENTED_EDGE ( 'NONE', *, *, #17146, .F. ) ;
#19627=ORIENTED_EDGE ( 'NONE', *, *, #10287, .F. ) ;
#19666=AXIS2_PLACEMENT_3D ( 'NONE', #19683, #14613, #32007 ) ;
#19683=CARTESIAN_POINT ( 'NONE',  ( 21.09785597605719332, 38.31023907818019580, 47.04930799450051637 ) ) ;
#19689=EDGE_LOOP ( 'NONE', ( #28299, #20612, #22908, #19607 ) ) ;
#19699=CARTESIAN_POINT ( 'NONE',  ( 21.09785597605718266, -13.49020584019834601, 105.1414762132873193 ) ) ;
#19719=DIRECTION ( 'NONE',  ( 0.000000000000000000, 0.000000000000000000, -1.000000000000000000 ) ) ;
#19720=CARTESIAN_POINT ( 'NONE',  ( -17.37805493069433282, -13.74047052604243646, 3.184189302845381153 ) ) ;
#19766=DIRECTION ( 'NONE',  ( 1.000000000000000000, 0.000000000000000000, 0.000000000000000000 ) ) ;
#19771=CARTESIAN_POINT ( 'NONE',  ( 21.09785597605719332, 7.881678200673685630, 47.04930799450051637 ) ) ;
#19772=TOROIDAL_SURFACE ( 'NONE', #6677, 83.95481021798164534, 94.94530576803560962 ) ;
#19796=DIRECTION ( 'NONE',  ( -0.000000000000000000, -1.000000000000000000, -0.000000000000000000 ) ) ;
#19798=DIRECTION ( 'NONE',  ( 0.000000000000000000, 0.000000000000000000, 1.000000000000000000 ) ) ;
#19815=CIRCLE ( 'NONE', #18742, 94.94530576803616384 ) ;
#19819=DIRECTION ( 'NONE',  ( 0.000000000000000000, 0.000000000000000000, -1.000000000000000000 ) ) ;
#19830=LINE ( 'NONE', #2447, #13910 ) ;
#19834=EDGE_LOOP ( 'NONE', ( #26414, #18146, #14619, #8042 ) ) ;
#19845=AXIS2_PLACEMENT_3D ( 'NONE', #19364, #32187, #27418 ) ;
#19859=ORIENTED_EDGE ( 'NONE', *, *, #15168, .F. ) ;
#19941=CYLINDRICAL_SURFACE ( 'NONE', #24028, 12.48414152717711900 ) ;
#19959=AXIS2_PLACEMENT_3D ( 'NONE', #29024, #6539, #26556 ) ;
#19965=CARTESIAN_POINT ( 'NONE',  ( 21.09785597605720042, -13.98292989133646103, 47.04930799450051637 ) ) ;
#19986=DIRECTION ( 'NONE',  ( 0.000000000000000000, 1.000000000000000000, -0.000000000000000000 ) ) ;
#19999=CIRCLE ( 'NONE', #1139, 19.21451602543517367 ) ;
#20020=VERTEX_POINT ( 'NONE', #6543 ) ;
#20034=AXIS2_PLACEMENT_3D ( 'NONE', #20550, #22850, #26242 ) ;
#20053=PRODUCT ( 'Membrane', 'Membrane', '', ( #30046 ) ) ;
#20065=ORIENTED_EDGE ( 'NONE', *, *, #31621, .F. ) ;
#20072=DIRECTION ( 'NONE',  ( 0.000000000000000000, 0.9550631830613039996, 0.2964022880492153122 ) ) ;
#20082=EDGE_CURVE ( 'NONE', #11143, #4372, #27082, .T. ) ;
#20088=ORIENTED_EDGE ( 'NONE', *, *, #32053, .T. ) ;
#20130=ORIENTED_EDGE ( 'NONE', *, *, #28609, .T. ) ;
#20158=ORIENTED_EDGE ( 'NONE', *, *, #13321, .F. ) ;
#20170=EDGE_LOOP ( 'NONE', ( #9521, #12469, #8310, #6261 ) ) ;
#20171=FACE_OUTER_BOUND ( 'NONE', #11339, .T. ) ;
#20173=ORIENTED_EDGE ( 'NONE', *, *, #7760, .F. ) ;
#20177=DIRECTION ( 'NONE',  ( 0.000000000000000000, 0.000000000000000000, -1.000000000000000000 ) ) ;
#20193=CIRCLE ( 'NONE', #22274, 0.2000000000000057288 ) ;
#20208=DIRECTION ( 'NONE',  ( 0.000000000000000000, 0.000000000000000000, -1.000000000000000000 ) ) ;
#20225=EDGE_LOOP ( 'NONE', ( #30842, #28259 ) ) ;
#20239=EDGE_CURVE ( 'NONE', #30184, #23467, #7718, .T. ) ;
#20312=CONICAL_SURFACE ( 'NONE', #14050, 55.69429210806286079, 1.269872874662818729 ) ;
#20328=CARTESIAN_POINT ( 'NONE',  ( 21.09785597605720042, -14.54791319078308653, 47.04930799450051637 ) ) ;
#20337=DIRECTION ( 'NONE',  ( -0.000000000000000000, -1.000000000000000000, -0.000000000000000000 ) ) ;
#20344=DIRECTION ( 'NONE',  ( -0.000000000000000000, -1.000000000000000000, -0.000000000000000000 ) ) ;
#20350=AXIS2_PLACEMENT_3D ( 'NONE', #21331, #30735, #23493 ) ;
#20362=FACE_OUTER_BOUND ( 'NONE', #3573, .T. ) ;
#20387=ORIENTED_EDGE ( 'NONE', *, *, #11379, .F. ) ;
#20389=EDGE_CURVE ( 'NONE', #17607, #24037, #11387, .T. ) ;
#20412=CARTESIAN_POINT ( 'NONE',  ( 21.09785597605720042, -14.04221034894631615, 47.04930799450051637 ) ) ;
#20458=DIRECTION ( 'NONE',  ( 0.000000000000000000, 0.000000000000000000, -1.000000000000000000 ) ) ;
#20469=CIRCLE ( 'NONE', #22020, 36.01080762834750715 ) ;
#20471=CARTESIAN_POINT ( 'NONE',  ( 21.09785597605719332, 7.237299147902269247, 66.50898490448155087 ) ) ;
#20550=CARTESIAN_POINT ( 'NONE',  ( 21.09785597605719332, 7.881678200673685630, 47.04930799450051637 ) ) ;
#20574=ORIENTED_EDGE ( 'NONE', *, *, #30218, .T. ) ;
#20587=VERTEX_POINT ( 'NONE', #29932 ) ;
#20595=CARTESIAN_POINT ( 'NONE',  ( 21.09785597605720042, -16.73545420775220194, -31.45069200549948363 ) ) ;
#20602=ORIENTED_EDGE ( 'NONE', *, *, #8665, .F. ) ;
#20603=AXIS2_PLACEMENT_3D ( 'NONE', #23860, #26813, #26327 ) ;
#20612=ORIENTED_EDGE ( 'NONE', *, *, #15263, .T. ) ;
#20636=CARTESIAN_POINT ( 'NONE',  ( 21.09785597605720042, -16.03545420775220265, 47.04930799450051637 ) ) ;
#20653=CARTESIAN_POINT ( 'NONE',  ( 21.09785597605718621, -13.49020584019834601, -11.04286022428629188 ) ) ;
#20662=AXIS2_PLACEMENT_3D ( 'NONE', #21687, #9228, #4302 ) ;
#20677=B_SPLINE_CURVE_WITH_KNOTS ( 'NONE', 3,
 ( #26285, #1486, #3792, #13817, #1327, #9210, #11348, #19201, #4113, #31541, #3959, #21674, #21335, #9046, #29228, #29066, #28918, #6587, #6742, #16581, #16740, #26767, #31698, #24137, #1655, #32020, #7237, #24628, #29566, #1977, #11998, #32190, #17232, #9542 ),
 .UNSPECIFIED., .F., .F.,
 ( 4, 2, 2, 2, 2, 2, 2, 2, 2, 2, 2, 2, 2, 2, 2, 2, 4 ),
 ( 0.000000000000000000, 0.03124999999999995837, 0.06249999999999994449, 0.09374999999999993061, 0.1249999999999999167, 0.1562499999999998890, 0.1874999999999998890, 0.2187499999999998612, 0.2499999999999998890, 0.2812499999999998890, 0.3124999999999998890, 0.3437499999999999445, 0.3749999999999999445, 0.4062499999999999445, 0.4374999999999999445, 0.4687500000000000000, 0.5000000000000000000 ),
 .UNSPECIFIED. ) ;
#20690=CARTESIAN_POINT ( 'NONE',  ( 6.626556088358251273, -13.30632128221581389, -6.978462942695593085 ) ) ;
#20704=VERTEX_POINT ( 'NONE', #26114 ) ;
#20717=AXIS2_PLACEMENT_3D ( 'NONE', #8635, #23724, #11260 ) ;
#20727=AXIS2_PLACEMENT_3D ( 'NONE', #6363, #4050, #29168 ) ;
#20777=EDGE_CURVE ( 'NONE', #12577, #25082, #5107, .T. ) ;
#20781=CARTESIAN_POINT ( 'NONE',  ( 21.09785597605720753, -13.64309448858209528, 105.9390803697710339 ) ) ;
#20809=VERTEX_POINT ( 'NONE', #32018 ) ;
#20825=ORIENTED_EDGE ( 'NONE', *, *, #13208, .T. ) ;
#20837=ORIENTED_EDGE ( 'NONE', *, *, #17792, .F. ) ;
#20844=EDGE_CURVE ( 'NONE', #8655, #7408, #19815, .T. ) ;
#20864=CARTESIAN_POINT ( 'NONE',  ( 49.06850489496600431, -13.30632128221581212, 95.48546547976138754 ) ) ;
#20867=DIRECTION ( 'NONE',  ( 0.000000000000000000, 0.000000000000000000, 1.000000000000000000 ) ) ;
#20877=AXIS2_PLACEMENT_3D ( 'NONE', #4303, #12014, #32040 ) ;
#20885=CARTESIAN_POINT ( 'NONE',  ( 21.09785597605719332, 17.36451738380053555, 47.04930799450051637 ) ) ;
#20889=CIRCLE ( 'NONE', #30863, 19.21451602543517367 ) ;
#20908=EDGE_LOOP ( 'NONE', ( #2234, #1093, #3942, #19546 ) ) ;
#20914=DIRECTION ( 'NONE',  ( 0.000000000000000000, 1.000000000000000000, -0.000000000000000000 ) ) ;
#20944=DIRECTION ( 'NONE',  ( 0.000000000000000000, 0.000000000000000000, -1.000000000000000000 ) ) ;
#20946=VERTEX_POINT ( 'NONE', #23776 ) ;
#20974=AXIS2_PLACEMENT_3D ( 'NONE', #31222, #8883, #10879 ) ;
#20975=ORIENTED_EDGE ( 'NONE', *, *, #6774, .F. ) ;
#21003=CARTESIAN_POINT ( 'NONE',  ( 6.626556088358270813, -13.30632128221581212, 101.0770789316966329 ) ) ;
#21004=CARTESIAN_POINT ( 'NONE',  ( 21.09785597605720042, -13.68834655544033652, -8.644984113562347972 ) ) ;
#21077=AXIS2_PLACEMENT_3D ( 'NONE', #8868, #18866, #1965 ) ;
#21084=DIRECTION ( 'NONE',  ( 0.000000000000000000, 0.000000000000000000, -1.000000000000000000 ) ) ;
#21097=DIRECTION ( 'NONE',  ( -1.000000000000000000, 0.000000000000000000, -1.224646799147353207E-16 ) ) ;
#21101=ORIENTED_EDGE ( 'NONE', *, *, #20844, .F. ) ;
#21105=ADVANCED_FACE ( 'NONE', ( #6320 ), #26087, .T. ) ;
#21159=CARTESIAN_POINT ( 'NONE',  ( -20.95081142018943510, -13.30632128221581389, 83.93193429851628196 ) ) ;
#21171=CARTESIAN_POINT ( 'NONE',  ( 24.75079866426202813, -13.30632128221581034, 102.8621610177830519 ) ) ;
#21178=DIRECTION ( 'NONE',  ( 0.000000000000000000, 0.000000000000000000, -1.000000000000000000 ) ) ;
#21194=ORIENTED_EDGE ( 'NONE', *, *, #226, .T. ) ;
#21202=CARTESIAN_POINT ( 'NONE',  ( 21.09785597605718976, 7.237299147902269247, 27.58963108451947832 ) ) ;
#21234=AXIS2_PLACEMENT_3D ( 'NONE', #20412, #28141, #5335 ) ;
#21283=DIRECTION ( 'NONE',  ( 0.000000000000000000, 0.000000000000000000, -1.000000000000000000 ) ) ;
#21291=AXIS2_PLACEMENT_3D ( 'NONE', #17936, #22861, #12870 ) ;
#21314=DIRECTION ( 'NONE',  ( -0.000000000000000000, -1.000000000000000000, -0.000000000000000000 ) ) ;
#21324=CARTESIAN_POINT ( 'NONE',  ( 21.09785597605720042, -13.59284023713420630, -8.674624342367264873 ) ) ;
#21331=CARTESIAN_POINT ( 'NONE',  ( 21.09785597605719332, -13.49020584019834601, 47.04930799450051637 ) ) ;
#21335=CARTESIAN_POINT ( 'NONE',  ( 73.43141673955736337, -13.74047052604243646, 21.24731629327111193 ) ) ;
#21389=AXIS2_PLACEMENT_3D ( 'NONE', #17566, #20344, #4940 ) ;
#21423=SHAPE_REPRESENTATION ( 'Membrane', ( #8172 ), #824 ) ;
#21471=ADVANCED_FACE ( 'NONE', ( #1832 ), #15955, .T. ) ;
#21479=TOROIDAL_SURFACE ( 'NONE', #20974, 78.39999999999999147, 0.1000000000000014350 ) ;
#21489=SPHERICAL_SURFACE ( 'NONE', #25957, 36.51080762834750715 ) ;
#21496=CIRCLE ( 'NONE', #18873, 58.70143199044622406 ) ;
#21498=EDGE_LOOP ( 'NONE', ( #23616, #24375, #23777, #26454 ) ) ;
#21502=ORIENTED_EDGE ( 'NONE', *, *, #24893, .F. ) ;
#21527=CARTESIAN_POINT ( 'NONE',  ( -22.76726271559795478, -13.74047052604243646, 8.573397087749011547 ) ) ;
#21547=EDGE_LOOP ( 'NONE', ( #2292, #31043, #15914, #16146 ) ) ;
#21553=EDGE_CURVE ( 'NONE', #9682, #14004, #1807, .T. ) ;
#21566=DIRECTION ( 'NONE',  ( 0.000000000000000000, 0.000000000000000000, -1.000000000000000000 ) ) ;
#21571=EDGE_CURVE ( 'NONE', #24849, #18606, #12838, .T. ) ;
#21582=DIRECTION ( 'NONE',  ( -0.000000000000000000, -1.000000000000000000, -0.000000000000000000 ) ) ;
#21587=ORIENTED_EDGE ( 'NONE', *, *, #14008, .T. ) ;
#21595=UNCERTAINTY_MEASURE_WITH_UNIT (LENGTH_MEASURE( 1.000000000000000082E-05 ), #17430, 'distance_accuracy_value', 'NONE');
#21649=ORIENTED_EDGE ( 'NONE', *, *, #23902, .T. ) ;
#21674=CARTESIAN_POINT ( 'NONE',  ( 71.62639656063520022, -13.74047052604243646, 17.87036105788319063 ) ) ;
#21678=CARTESIAN_POINT ( 'NONE',  ( 21.09785597605719332, 77.37245976740706510, -36.90550222348115028 ) ) ;
#21680=ORIENTED_EDGE ( 'NONE', *, *, #12621, .T. ) ;
#21687=CARTESIAN_POINT ( 'NONE',  ( 21.09785597605720042, -13.88867167006704939, 47.04930799450051637 ) ) ;
#21701=DIRECTION ( 'NONE',  ( 1.000000000000000000, 0.000000000000000000, 0.000000000000000000 ) ) ;
#21716=CARTESIAN_POINT ( 'NONE',  ( 21.09785597605720753, -16.03545420775220265, 117.6483275080933169 ) ) ;
#21744=DIRECTION ( 'NONE',  ( 1.000000000000000000, 0.000000000000000000, 0.000000000000000000 ) ) ;
#21745=DIRECTION ( 'NONE',  ( 0.000000000000000000, 0.000000000000000000, -1.000000000000000000 ) ) ;
#21751=VERTEX_POINT ( 'NONE', #5278 ) ;
#21807=EDGE_CURVE ( 'NONE', #15416, #31613, #8377, .T. ) ;
#21829=DIRECTION ( 'NONE',  ( -0.000000000000000000, -1.000000000000000000, -0.000000000000000000 ) ) ;
#21845=CARTESIAN_POINT ( 'NONE',  ( 21.09785597605721108, -17.03545420775220265, 125.4493079945005150 ) ) ;
#21937=AXIS2_PLACEMENT_3D ( 'NONE', #1942, #29038, #32433 ) ;
#21957=ADVANCED_FACE ( 'NONE', ( #24597 ), #9019, .F. ) ;
#21962=EDGE_CURVE ( 'NONE', #15585, #26708, #14426, .T. ) ;
#21973=EDGE_LOOP ( 'NONE', ( #3360, #7119, #26597, #31686 ) ) ;
#21975=DIRECTION ( 'NONE',  ( 0.000000000000000000, 0.000000000000000000, 1.000000000000000000 ) ) ;
#21982=CARTESIAN_POINT ( 'NONE',  ( 76.55093444394998414, -13.30632128221581212, 39.74351294429737180 ) ) ;
#22015=CARTESIAN_POINT ( 'NONE',  ( -36.75072804420383221, -13.74047052604243646, 54.67070450616914457 ) ) ;
#22020=AXIS2_PLACEMENT_3D ( 'NONE', #14537, #2054, #21744 ) ;
#22037=AXIS2_PLACEMENT_3D ( 'NONE', #28421, #27769, #15298 ) ;
#22044=CIRCLE ( 'NONE', #17326, 0.09999999999998898659 ) ;
#22064=CARTESIAN_POINT ( 'NONE',  ( 21.09785597605720042, -17.03545420775220265, 47.04930799450051637 ) ) ;
#22068=CARTESIAN_POINT ( 'NONE',  ( 21.09785597605719332, 17.36451738380053555, 47.04930799450051637 ) ) ;
#22080=EDGE_CURVE ( 'NONE', #20020, #8655, #19830, .T. ) ;
#22097=CARTESIAN_POINT ( 'NONE',  ( 21.09785597605720042, -13.56320000832927875, 102.6777340130621639 ) ) ;
#22101=DIRECTION ( 'NONE',  ( 0.000000000000000000, 0.000000000000000000, -1.000000000000000000 ) ) ;
#22121=ORIENTED_EDGE ( 'NONE', *, *, #30755, .F. ) ;
#22129=CIRCLE ( 'NONE', #17428, 12.98419020052701889 ) ;
#22153=ADVANCED_FACE ( 'NONE', ( #23279 ), #27515, .T. ) ;
#22159=ORIENTED_EDGE ( 'NONE', *, *, #22863, .F. ) ;
#22168=AXIS2_PLACEMENT_3D ( 'NONE', #27203, #4727, #128 ) ;
#22242=EDGE_LOOP ( 'NONE', ( #17057, #31262, #23228, #7400 ) ) ;
#22247=CIRCLE ( 'NONE', #8115, 12.98419020052702599 ) ;
#22249=CIRCLE ( 'NONE', #7614, 58.84990142703892246 ) ;
#22272=DIRECTION ( 'NONE',  ( 0.000000000000000000, 0.000000000000000000, 1.000000000000000000 ) ) ;
#22274=AXIS2_PLACEMENT_3D ( 'NONE', #14447, #17378, #6892 ) ;
#22305=DIRECTION ( 'NONE',  ( -0.000000000000000000, -1.000000000000000000, -0.000000000000000000 ) ) ;
#22308=ORIENTED_EDGE ( 'NONE', *, *, #1166, .F. ) ;
#22325=CARTESIAN_POINT ( 'NONE',  ( 21.09785597605720753, -13.87844638871996850, 106.4909947499981513 ) ) ;
#22340=DIRECTION ( 'NONE',  ( 0.000000000000000000, 0.000000000000000000, -1.000000000000000000 ) ) ;
#22362=VERTEX_POINT ( 'NONE', #26693 ) ;
#22376=EDGE_CURVE ( 'NONE', #20809, #11333, #25079, .T. ) ;
#22391=DIRECTION ( 'NONE',  ( 0.000000000000000000, 0.000000000000000000, -1.000000000000000000 ) ) ;
#22406=AXIS2_PLACEMENT_3D ( 'NONE', #5851, #18140, #21084 ) ;
#22432=ORIENTED_EDGE ( 'NONE', *, *, #9028, .F. ) ;
#22456=CIRCLE ( 'NONE', #8331, 69.59901951359279337 ) ;
#22457=DIRECTION ( 'NONE',  ( 0.000000000000000000, 0.000000000000000000, -1.000000000000000000 ) ) ;
#22479=DIRECTION ( 'NONE',  ( -1.000000000000000000, 0.000000000000000000, -1.224646799147353207E-16 ) ) ;
#22489=ORIENTED_EDGE ( 'NONE', *, *, #8083, .F. ) ;
#22538=AXIS2_PLACEMENT_3D ( 'NONE', #12712, #32238, #4652 ) ;
#22544=ORIENTED_EDGE ( 'NONE', *, *, #21553, .T. ) ;
#22549=CARTESIAN_POINT ( 'NONE',  ( 33.88204617658421824, 17.36451738380053555, 47.04930799450051637 ) ) ;
#22563=TOROIDAL_SURFACE ( 'NONE', #6332, 83.95485889133257729, 94.44530576803552435 ) ;
#22565=EDGE_CURVE ( 'NONE', #16711, #15162, #8299, .T. ) ;
#22639=AXIS2_PLACEMENT_3D ( 'NONE', #31473, #8981, #24235 ) ;
#22645=ORIENTED_EDGE ( 'NONE', *, *, #22896, .F. ) ;
#22655=AXIS2_PLACEMENT_3D ( 'NONE', #29143, #16649, #3703 ) ;
#22659=VERTEX_POINT ( 'NONE', #8770 ) ;
#22683=TOROIDAL_SURFACE ( 'NONE', #14820, 55.72393233686778302, 0.09999999999999760469 ) ;
#22760=ORIENTED_EDGE ( 'NONE', *, *, #12061, .F. ) ;
#22769=FACE_OUTER_BOUND ( 'NONE', #17497, .T. ) ;
#22786=DIRECTION ( 'NONE',  ( 0.000000000000000000, 0.000000000000000000, 1.000000000000000000 ) ) ;
#22796=CIRCLE ( 'NONE', #260, 58.67217910650386870 ) ;
#22812=ORIENTED_EDGE ( 'NONE', *, *, #21553, .F. ) ;
#22844=AXIS2_PLACEMENT_3D ( 'NONE', #22549, #2857, #12893 ) ;
#22850=DIRECTION ( 'NONE',  ( 0.000000000000000000, 1.000000000000000000, -0.000000000000000000 ) ) ;
#22851=DIRECTION ( 'NONE',  ( 0.000000000000000000, 1.000000000000000000, -0.000000000000000000 ) ) ;
#22861=DIRECTION ( 'NONE',  ( -1.000000000000000000, 0.000000000000000000, 0.000000000000000000 ) ) ;
#22863=EDGE_CURVE ( 'NONE', #24037, #24849, #30861, .T. ) ;
#22870=DIRECTION ( 'NONE',  ( 0.000000000000000000, 0.000000000000000000, -1.000000000000000000 ) ) ;
#22880=CARTESIAN_POINT ( 'NONE',  ( 21.09785597605719332, -13.49020584019834601, 47.04930799450051637 ) ) ;
#22891=ORIENTED_EDGE ( 'NONE', *, *, #6257, .F. ) ;
#22896=EDGE_CURVE ( 'NONE', #6923, #7408, #26369, .T. ) ;
#22908=ORIENTED_EDGE ( 'NONE', *, *, #19559, .T. ) ;
#22911=FACE_OUTER_BOUND ( 'NONE', #27208, .T. ) ;
#22931=ORIENTED_EDGE ( 'NONE', *, *, #29533, .F. ) ;
#22993=DIRECTION ( 'NONE',  ( 0.000000000000000000, 1.000000000000000000, -0.000000000000000000 ) ) ;
#22995=CARTESIAN_POINT ( 'NONE',  ( 21.09785597605719332, 34.11266481626051217, 47.04930799450051637 ) ) ;
#22999=SURFACE_STYLE_FILL_AREA ( #42 ) ;
#23008=EDGE_LOOP ( 'NONE', ( #5757, #9480, #12148, #20173 ) ) ;
#23061=ORIENTED_EDGE ( 'NONE', *, *, #6004, .F. ) ;
#23089=DIRECTION ( 'NONE',  ( 0.000000000000000000, 0.000000000000000000, -1.000000000000000000 ) ) ;
#23095=CARTESIAN_POINT ( 'NONE',  ( 21.09785597605719332, 6.574714862014670480, 67.18583656269663607 ) ) ;
#23120=ORIENTED_EDGE ( 'NONE', *, *, #20777, .T. ) ;
#23124=ADVANCED_FACE ( 'NONE', ( #12302 ), #15673, .F. ) ;
#23128=CARTESIAN_POINT ( 'NONE',  ( 21.09785597605719332, 15.24673779880127178, 47.04930799450051637 ) ) ;
#23138=CIRCLE ( 'NONE', #87, 5.499019513592787511 ) ;
#23149=DIRECTION ( 'NONE',  ( 0.000000000000000000, -0.2964022880492245271, -0.9550631830613013351 ) ) ;
#23154=CARTESIAN_POINT ( 'NONE',  ( 17.44491328785239048, -13.30632128221581034, 102.8621610177830519 ) ) ;
#23160=DIRECTION ( 'NONE',  ( 0.000000000000000000, 0.000000000000000000, -1.000000000000000000 ) ) ;
#23167=ADVANCED_FACE ( 'NONE', ( #10492 ), #10440, .F. ) ;
#23170=EDGE_LOOP ( 'NONE', ( #6307, #2607, #3074, #26915 ) ) ;
#23177=VERTEX_POINT ( 'NONE', #32488 ) ;
#23206=DIRECTION ( 'NONE',  ( -1.000000000000000000, 0.000000000000000000, 0.000000000000000000 ) ) ;
#23228=ORIENTED_EDGE ( 'NONE', *, *, #25318, .T. ) ;
#23232=CIRCLE ( 'NONE', #14328, 13.23540278830031447 ) ;
#23241=TOROIDAL_SURFACE ( 'NONE', #30590, 55.78321279447762748, 0.1000000000000016986 ) ;
#23252=DIRECTION ( 'NONE',  ( 0.000000000000000000, 0.000000000000000000, -1.000000000000000000 ) ) ;
#23279=FACE_OUTER_BOUND ( 'NONE', #1117, .T. ) ;
#23300=VECTOR ( 'NONE', #23149, 999.9999999999998863 ) ;
#23327=CARTESIAN_POINT ( 'NONE',  ( 21.09785597605720042, -16.63545420775220407, 47.04930799450051637 ) ) ;
#23335=CARTESIAN_POINT ( 'NONE',  ( 74.06012918148381630, -13.30632128221581567, 65.03308317646937553 ) ) ;
#23338=EDGE_LOOP ( 'NONE', ( #20574, #21194, #24378, #10930 ) ) ;
#23346=AXIS2_PLACEMENT_3D ( 'NONE', #23886, #7096, #7435 ) ;
#23356=AXIS2_PLACEMENT_3D ( 'NONE', #32450, #17506, #31793 ) ;
#23364=DIRECTION ( 'NONE',  ( -0.000000000000000000, -1.000000000000000000, -0.000000000000000000 ) ) ;
#23365=DIRECTION ( 'NONE',  ( 0.000000000000000000, 1.000000000000000000, -0.000000000000000000 ) ) ;
#23425=DIRECTION ( 'NONE',  ( 0.000000000000000000, 0.000000000000000000, -1.000000000000000000 ) ) ;
#23426=ORIENTED_EDGE ( 'NONE', *, *, #21962, .T. ) ;
#23437=DIRECTION ( 'NONE',  ( 0.000000000000000000, -1.000000000000000000, 0.000000000000000000 ) ) ;
#23442=ORIENTED_EDGE ( 'NONE', *, *, #4905, .T. ) ;
#23467=VERTEX_POINT ( 'NONE', #268 ) ;
#23481=EDGE_LOOP ( 'NONE', ( #17985, #21680, #8256, #24443 ) ) ;
#23493=DIRECTION ( 'NONE',  ( 0.000000000000000000, 0.000000000000000000, -1.000000000000000000 ) ) ;
#23596=EDGE_LOOP ( 'NONE', ( #214, #20065, #13085, #17402 ) ) ;
#23616=ORIENTED_EDGE ( 'NONE', *, *, #16733, .F. ) ;
#23631=AXIS2_PLACEMENT_3D ( 'NONE', #10756, #28304, #1047 ) ;
#23641=CARTESIAN_POINT ( 'NONE',  ( -23.27936906821728158, -13.30632128221581212, 81.09457859485948461 ) ) ;
#23662=DIRECTION ( 'NONE',  ( 0.000000000000000000, 1.000000000000000000, 0.000000000000000000 ) ) ;
#23679=ORIENTED_EDGE ( 'NONE', *, *, #10285, .T. ) ;
#23693=DIRECTION ( 'NONE',  ( -0.000000000000000000, -1.000000000000000000, -0.000000000000000000 ) ) ;
#23707=VERTEX_POINT ( 'NONE', #1549 ) ;
#23710=ORIENTED_EDGE ( 'NONE', *, *, #23938, .T. ) ;
#23715=DIRECTION ( 'NONE',  ( -1.224646799147353207E-16, 0.000000000000000000, 1.000000000000000000 ) ) ;
#23724=DIRECTION ( 'NONE',  ( -0.000000000000000000, -1.000000000000000000, -0.000000000000000000 ) ) ;
#23735=CARTESIAN_POINT ( 'NONE',  ( 21.09785597605720042, -16.03545420775220265, 47.04930799450051637 ) ) ;
#23750=APPLICATION_CONTEXT ( 'automotive_design' ) ;
#23761=DIRECTION ( 'NONE',  ( 0.000000000000000000, 1.000000000000000000, -0.000000000000000000 ) ) ;
#23776=CARTESIAN_POINT ( 'NONE',  ( 21.09785597605718266, 14.77310068074637961, 60.28471078280082907 ) ) ;
#23777=ORIENTED_EDGE ( 'NONE', *, *, #6028, .T. ) ;
#23806=FACE_OUTER_BOUND ( 'NONE', #18535, .T. ) ;
#23821=TOROIDAL_SURFACE ( 'NONE', #8121, 70.59901951359279337, 0.6000000000000020872 ) ;
#23830=DIRECTION ( 'NONE',  ( 0.000000000000000000, 1.000000000000000000, -0.000000000000000000 ) ) ;
#23843=TOROIDAL_SURFACE ( 'NONE', #9709, 13.48414152717812797, 1.000000000001010525 ) ;
#23847=CARTESIAN_POINT ( 'NONE',  ( 21.09785597605720753, -13.37218737171702543, -8.638398481670979123 ) ) ;
#23860=CARTESIAN_POINT ( 'NONE',  ( 21.09785597605720042, -13.98292989133646103, 47.04930799450051637 ) ) ;
#23867=AXIS2_PLACEMENT_3D ( 'NONE', #21324, #19027, #26430 ) ;
#23886=CARTESIAN_POINT ( 'NONE',  ( 21.09785597605719332, 6.671061906060458568, 47.04930799450051637 ) ) ;
#23902=EDGE_CURVE ( 'NONE', #24243, #29052, #25169, .T. ) ;
#23923=CIRCLE ( 'NONE', #21291, 0.1000000000000028644 ) ;
#23933=DIRECTION ( 'NONE',  ( 0.000000000000000000, 0.000000000000000000, 1.000000000000000000 ) ) ;
#23938=EDGE_CURVE ( 'NONE', #18375, #20946, #31950, .T. ) ;
#23947=DIRECTION ( 'NONE',  ( -1.000000000000000000, 0.000000000000000000, -1.926892052941620175E-16 ) ) ;
#23950=ORIENTED_EDGE ( 'NONE', *, *, #17621, .F. ) ;
#23955=EDGE_LOOP ( 'NONE', ( #30989, #19460, #32310, #2974, #3501 ) ) ;
#23965=CARTESIAN_POINT ( 'NONE',  ( 45.83138912416442423, -13.30632128221581212, -3.117123918615745115 ) ) ;
#23968=EDGE_CURVE ( 'NONE', #28177, #26439, #2628, .T. ) ;
#24021=DIRECTION ( 'NONE',  ( 0.000000000000000000, 0.000000000000000000, -1.000000000000000000 ) ) ;
#24027=AXIS2_PLACEMENT_3D ( 'NONE', #15944, #1322, #25948 ) ;
#24028=AXIS2_PLACEMENT_3D ( 'NONE', #29804, #2060, #7317 ) ;
#24029=CYLINDRICAL_SURFACE ( 'NONE', #4534, 12.98419020052702599 ) ;
#24036=DIRECTION ( 'NONE',  ( -0.000000000000000000, -1.000000000000000000, -0.000000000000000000 ) ) ;
#24037=VERTEX_POINT ( 'NONE', #722 ) ;
#24055=DIRECTION ( 'NONE',  ( 0.000000000000000000, 1.000000000000000000, -0.000000000000000000 ) ) ;
#24057=CIRCLE ( 'NONE', #30892, 12.48414152717711190 ) ;
#24062=EDGE_LOOP ( 'NONE', ( #19085, #17648, #22645, #22891 ) ) ;
#24074=DIRECTION ( 'NONE',  ( 0.000000000000000000, 1.000000000000000000, -0.000000000000000000 ) ) ;
#24099=ORIENTED_EDGE ( 'NONE', *, *, #18618, .F. ) ;
#24110=EDGE_LOOP ( 'NONE', ( #1760, #4712, #30534, #25485 ) ) ;
#24115=EDGE_CURVE ( 'NONE', #9682, #23707, #3675, .T. ) ;
#24121=ORIENTED_EDGE ( 'NONE', *, *, #22565, .F. ) ;
#24137=CARTESIAN_POINT ( 'NONE',  ( 67.39212317433587884, -13.74047052604243646, 82.56529288175445913 ) ) ;
#24142=TOROIDAL_SURFACE ( 'NONE', #10002, 55.72393233686778302, 0.09999999999999760469 ) ;
#24147=DIRECTION ( 'NONE',  ( -0.000000000000000000, 0.000000000000000000, -1.000000000000000000 ) ) ;
#24153=EDGE_CURVE ( 'NONE', #29601, #8764, #6302, .T. ) ;
#24215=DIRECTION ( 'NONE',  ( 0.000000000000000000, 0.000000000000000000, -1.000000000000000000 ) ) ;
#24216=CARTESIAN_POINT ( 'NONE',  ( 21.09785597605720753, -13.88867167006704939, 105.7507399849467475 ) ) ;
#24225=TOROIDAL_SURFACE ( 'NONE', #27372, 58.88977237527051756, 0.5999999999999987566 ) ;
#24235=DIRECTION ( 'NONE',  ( 0.000000000000000000, 0.000000000000000000, -1.000000000000000000 ) ) ;
#24239=CIRCLE ( 'NONE', #12193, 55.62842601856165459 ) ;
#24243=VERTEX_POINT ( 'NONE', #31402 ) ;
#24245=ORIENTED_EDGE ( 'NONE', *, *, #15400, .F. ) ;
#24250=FACE_BOUND ( 'NONE', #9803, .T. ) ;
#24256=VERTEX_POINT ( 'NONE', #30082 ) ;
#24259=CARTESIAN_POINT ( 'NONE',  ( 21.09785597605719332, 7.237299147902269247, 47.04930799450051637 ) ) ;
#24272=CIRCLE ( 'NONE', #6983, 12.48414152717711900 ) ;
#24281=ORIENTED_EDGE ( 'NONE', *, *, #15853, .T. ) ;
#24288=SPHERICAL_SURFACE ( 'NONE', #19666, 36.01080762834750715 ) ;
#24293=ORIENTED_EDGE ( 'NONE', *, *, #29533, .T. ) ;
#24299=FACE_OUTER_BOUND ( 'NONE', #21973, .T. ) ;
#24313=DIRECTION ( 'NONE',  ( 0.000000000000000000, 0.000000000000000000, 1.000000000000000000 ) ) ;
#24322=CARTESIAN_POINT ( 'NONE',  ( -31.23570478744295542, -13.74047052604243646, 72.85129969572992081 ) ) ;
#24359=AXIS2_PLACEMENT_3D ( 'NONE', #2318, #10036, #29570 ) ;
#24375=ORIENTED_EDGE ( 'NONE', *, *, #24855, .F. ) ;
#24378=ORIENTED_EDGE ( 'NONE', *, *, #4882, .F. ) ;
#24396=CYLINDRICAL_SURFACE ( 'NONE', #22639, 78.50000000000000000 ) ;
#24410=FACE_OUTER_BOUND ( 'NONE', #9093, .T. ) ;
#24417=ORIENTED_EDGE ( 'NONE', *, *, #15802, .F. ) ;
#24443=ORIENTED_EDGE ( 'NONE', *, *, #11928, .F. ) ;
#24459=CARTESIAN_POINT ( 'NONE',  ( 21.09785597605720042, -16.63545420775220407, 47.04930799450051637 ) ) ;
#24480=ADVANCED_FACE ( 'NONE', ( #5292 ), #8439, .T. ) ;
#24497=DIRECTION ( 'NONE',  ( 0.000000000000000000, 0.000000000000000000, -1.000000000000000000 ) ) ;
#24513=DIRECTION ( 'NONE',  ( -0.000000000000000000, -1.000000000000000000, -0.000000000000000000 ) ) ;
#24556=FACE_OUTER_BOUND ( 'NONE', #20908, .T. ) ;
#24560=ADVANCED_FACE ( 'NONE', ( #24410 ), #4760, .F. ) ;
#24597=FACE_OUTER_BOUND ( 'NONE', #17050, .T. ) ;
#24599=CARTESIAN_POINT ( 'NONE',  ( 21.09785597605717911, -12.82881809906321813, 103.0103621606812681 ) ) ;
#24628=CARTESIAN_POINT ( 'NONE',  ( 50.27680291267451906, -13.74047052604243468, 97.57784857907853393 ) ) ;
#24633=CIRCLE ( 'NONE', #12608, 55.62393233686778160 ) ;
#24637=VECTOR ( 'NONE', #20072, 1000.000000000000227 ) ;
#24670=LINE ( 'NONE', #12860, #6279 ) ;
#24675=CARTESIAN_POINT ( 'NONE',  ( 21.09785597605718976, 1.799431449832689101, 47.04930799450051637 ) ) ;
#24690=AXIS2_PLACEMENT_3D ( 'NONE', #19606, #29637, #4681 ) ;
#24700=CARTESIAN_POINT ( 'NONE',  ( 21.09785597605720042, -13.59284023713420630, 47.04930799450051637 ) ) ;
#24702=DIRECTION ( 'NONE',  ( 0.000000000000000000, 0.000000000000000000, -1.000000000000000000 ) ) ;
#24703=CARTESIAN_POINT ( 'NONE',  ( 21.09785597605721108, -16.73545420775220194, 125.4493079945005150 ) ) ;
#24765=AXIS2_PLACEMENT_3D ( 'NONE', #25303, #30388, #2167 ) ;
#24769=ORIENTED_EDGE ( 'NONE', *, *, #14847, .T. ) ;
#24790=ORIENTED_EDGE ( 'NONE', *, *, #13208, .F. ) ;
#24794=ORIENTED_EDGE ( 'NONE', *, *, #23968, .F. ) ;
#24833=CARTESIAN_POINT ( 'NONE',  ( 21.09785597605719332, 15.43591091851532759, 33.06511779397247608 ) ) ;
#24845=VECTOR ( 'NONE', #17942, 1000.000000000000000 ) ;
#24849=VERTEX_POINT ( 'NONE', #29124 ) ;
#24852=EDGE_CURVE ( 'NONE', #14823, #29876, #6640, .T. ) ;
#24855=EDGE_CURVE ( 'NONE', #29052, #24243, #70, .T. ) ;
#24889=CIRCLE ( 'NONE', #24359, 12.68414152717711119 ) ;
#24893=EDGE_CURVE ( 'NONE', #14245, #27708, #9755, .T. ) ;
#24930=TOROIDAL_SURFACE ( 'NONE', #20727, 12.68414152717710763, 0.1999999999999992339 ) ;
#24931=EDGE_LOOP ( 'NONE', ( #25688, #1866, #10761, #9208, #18083 ) ) ;
#24940=DIRECTION ( 'NONE',  ( 0.000000000000000000, 1.000000000000000000, -0.000000000000000000 ) ) ;
#24951=CARTESIAN_POINT ( 'NONE',  ( 21.09785597605720042, -14.03534765547855656, -12.76032168114853782 ) ) ;
#24979=EDGE_CURVE ( 'NONE', #23177, #18054, #15330, .T. ) ;
#24991=ADVANCED_FACE ( 'NONE', ( #8080 ), #28101, .T. ) ;
#25062=ORIENTED_EDGE ( 'NONE', *, *, #6028, .F. ) ;
#25075=DIRECTION ( 'NONE',  ( 0.000000000000000000, 1.000000000000000000, -0.000000000000000000 ) ) ;
#25079=CIRCLE ( 'NONE', #6702, 55.62842601856165459 ) ;
#25082=VERTEX_POINT ( 'NONE', #14976 ) ;
#25106=AXIS2_PLACEMENT_3D ( 'NONE', #24459, #21829, #1817 ) ;
#25108=DIRECTION ( 'NONE',  ( 0.000000000000000000, 0.000000000000000000, -1.000000000000000000 ) ) ;
#25149=ORIENTED_EDGE ( 'NONE', *, *, #9258, .T. ) ;
#25169=CIRCLE ( 'NONE', #2074, 59.80962967564905597 ) ;
#25204=DIRECTION ( 'NONE',  ( -1.000000000000000000, 0.000000000000000000, 0.000000000000000000 ) ) ;
#25214=EDGE_CURVE ( 'NONE', #21751, #6567, #19999, .T. ) ;
#25234=CARTESIAN_POINT ( 'NONE',  ( 21.09785597605720042, -13.64309448858209528, 47.04930799450051637 ) ) ;
#25285=EDGE_LOOP ( 'NONE', ( #21101, #28969, #29355, #8195 ) ) ;
#25303=CARTESIAN_POINT ( 'NONE',  ( 21.09785597605719332, 15.24673779880127356, 60.53344952167864790 ) ) ;
#25304=EDGE_CURVE ( 'NONE', #14245, #23467, #31025, .T. ) ;
#25318=EDGE_CURVE ( 'NONE', #9202, #31146, #28403, .T. ) ;
#25322=ORIENTED_EDGE ( 'NONE', *, *, #12573, .T. ) ;
#25349=PLANE ( 'NONE',  #22844 ) ;
#25351=DIRECTION ( 'NONE',  ( 0.000000000000000000, 0.000000000000000000, -1.000000000000000000 ) ) ;
#25369=CIRCLE ( 'NONE', #17492, 0.1000000000000028644 ) ;
#25373=AXIS2_PLACEMENT_3D ( 'NONE', #29878, #5085, #7059 ) ;
#25397=ADVANCED_FACE ( 'NONE', ( #15218 ), #14249, .T. ) ;
#25447=ADVANCED_FACE ( 'NONE', ( #30802 ), #28922, .T. ) ;
#25448=AXIS2_PLACEMENT_3D ( 'NONE', #16212, #6535, #11148 ) ;
#25451=AXIS2_PLACEMENT_3D ( 'NONE', #11895, #24036, #6808 ) ;
#25463=PLANE ( 'NONE',  #13787 ) ;
#25485=ORIENTED_EDGE ( 'NONE', *, *, #5597, .F. ) ;
#25497=ORIENTED_EDGE ( 'NONE', *, *, #12628, .T. ) ;
#25525=ORIENTED_EDGE ( 'NONE', *, *, #30185, .T. ) ;
#25530=ADVANCED_FACE ( 'NONE', ( #6331 ), #2204, .F. ) ;
#25547=DIRECTION ( 'NONE',  ( -0.000000000000000000, -1.000000000000000000, -0.000000000000000000 ) ) ;
#25603=ORIENTED_EDGE ( 'NONE', *, *, #27393, .T. ) ;
#25606=ORIENTED_EDGE ( 'NONE', *, *, #11094, .F. ) ;
#25607=AXIS2_PLACEMENT_3D ( 'NONE', #14788, #11672, #7230 ) ;
#25610=EDGE_CURVE ( 'NONE', #23467, #22362, #29482, .T. ) ;
#25649=ORIENTED_EDGE ( 'NONE', *, *, #24852, .T. ) ;
#25673=LINE ( 'NONE', #7968, #11060 ) ;
#25688=ORIENTED_EDGE ( 'NONE', *, *, #9426, .F. ) ;
#25723=DIRECTION ( 'NONE',  ( 1.000000000000000000, 0.000000000000000000, -1.224646799147353207E-16 ) ) ;
#25727=DIRECTION ( 'NONE',  ( 0.000000000000000000, 1.000000000000000000, -0.000000000000000000 ) ) ;
#25769=ORIENTED_EDGE ( 'NONE', *, *, #10097, .F. ) ;
#25788=EDGE_LOOP ( 'NONE', ( #5888, #18918, #18605, #10347 ) ) ;
#25790=CARTESIAN_POINT ( 'NONE',  ( 69.53401346131808225, -13.30632128221581567, 75.01995691340934513 ) ) ;
#25811=CARTESIAN_POINT ( 'NONE',  ( 21.09785597605719332, 34.11266481626051217, 59.53344952167763182 ) ) ;
#25836=ORIENTED_EDGE ( 'NONE', *, *, #15628, .F. ) ;
#25842=CIRCLE ( 'NONE', #15355, 0.9999999999999991118 ) ;
#25846=EDGE_LOOP ( 'NONE', ( #2596, #25649, #10303, #29462 ) ) ;
#25927=TOROIDAL_SURFACE ( 'NONE', #26988, 83.95485889133257729, 94.44530576803552435 ) ;
#25939=DIRECTION ( 'NONE',  ( -1.000000000000000000, 0.000000000000000000, -1.224646799147353207E-16 ) ) ;
#25942=CARTESIAN_POINT ( 'NONE',  ( 21.09785597605719332, 14.58544108513610027, 47.04930799450051637 ) ) ;
#25948=DIRECTION ( 'NONE',  ( 0.000000000000000000, 0.000000000000000000, -1.000000000000000000 ) ) ;
#25957=AXIS2_PLACEMENT_3D ( 'NONE', #6576, #16568, #6730 ) ;
#25974=DIRECTION ( 'NONE',  ( 0.000000000000000000, 0.000000000000000000, -1.000000000000000000 ) ) ;
#25977=TOROIDAL_SURFACE ( 'NONE', #21234, 58.86319174311611846, 0.1999999999999984290 ) ;
#25981=DIRECTION ( 'NONE',  ( 0.000000000000000000, 0.000000000000000000, -1.000000000000000000 ) ) ;
#25999=EDGE_LOOP ( 'NONE', ( #6869, #3974, #6976, #1723 ) ) ;
#26004=MECHANICAL_DESIGN_GEOMETRIC_PRESENTATION_REPRESENTATION('',(#19174),#18655);
#26032=DIRECTION ( 'NONE',  ( 0.000000000000000000, 0.000000000000000000, -1.000000000000000000 ) ) ;
#26046=AXIS2_PLACEMENT_3D ( 'NONE', #14748, #25075, #2588 ) ;
#26048=CARTESIAN_POINT ( 'NONE',  ( 21.09785597605719332, 17.16451738380053271, 47.04930799450051637 ) ) ;
#26064=DIRECTION ( 'NONE',  ( 0.000000000000000000, 1.000000000000000000, -0.000000000000000000 ) ) ;
#26066=ORIENTED_EDGE ( 'NONE', *, *, #6481, .T. ) ;
#26087=TOROIDAL_SURFACE ( 'NONE', #22406, 55.72393233686778302, 0.09999999999999760469 ) ;
#26089=DIRECTION ( 'NONE',  ( 0.000000000000000000, 0.000000000000000000, -1.000000000000000000 ) ) ;
#26114=CARTESIAN_POINT ( 'NONE',  ( 21.09785597605719332, 17.16451738380053271, 60.03349819502753348 ) ) ;
#26143=DIRECTION ( 'NONE',  ( 1.000000000000000000, 0.000000000000000000, -1.224646799147353207E-16 ) ) ;
#26149=LINE ( 'NONE', #23847, #32366 ) ;
#26188=AXIS2_PLACEMENT_3D ( 'NONE', #21678, #9546, #7240 ) ;
#26214=AXIS2_PLACEMENT_3D ( 'NONE', #30843, #30688, #2936 ) ;
#26219=DIRECTION ( 'NONE',  ( -0.000000000000000000, -1.000000000000000000, -0.000000000000000000 ) ) ;
#26238=DIRECTION ( 'NONE',  ( 0.000000000000000000, 0.000000000000000000, -1.000000000000000000 ) ) ;
#26242=DIRECTION ( 'NONE',  ( 0.000000000000000000, 0.000000000000000000, -1.000000000000000000 ) ) ;
#26248=CARTESIAN_POINT ( 'NONE',  ( 40.31237200149237765, 7.264443105416139801, 47.04930799450051637 ) ) ;
#26250=CIRCLE ( 'NONE', #27831, 12.68414152717711119 ) ;
#26257=EDGE_CURVE ( 'NONE', #6352, #10039, #3603, .T. ) ;
#26263=CARTESIAN_POINT ( 'NONE',  ( -29.06857593705904819, -13.30632128221580857, 22.31577484639326769 ) ) ;
#26276=AXIS2_PLACEMENT_3D ( 'NONE', #7960, #23206, #17953 ) ;
#26279=CARTESIAN_POINT ( 'NONE',  ( 21.09785597605719687, -13.30631372918550959, -8.763520691563154941 ) ) ;
#26285=CARTESIAN_POINT ( 'NONE',  ( 21.09785597605719332, -13.74048473023143835, -11.17459240385188934 ) ) ;
#26292=AXIS2_PLACEMENT_3D ( 'NONE', #5691, #25547, #23252 ) ;
#26294=ADVANCED_FACE ( 'NONE', ( #23806 ), #27721, .T. ) ;
#26324=DIRECTION ( 'NONE',  ( 0.000000000000000000, 1.000000000000000000, -0.000000000000000000 ) ) ;
#26327=DIRECTION ( 'NONE',  ( 0.000000000000000000, 0.000000000000000000, 1.000000000000000000 ) ) ;
#26329=FACE_OUTER_BOUND ( 'NONE', #30140, .T. ) ;
#26334=CIRCLE ( 'NONE', #20034, 19.25826962553310295 ) ;
#26369=B_SPLINE_CURVE_WITH_KNOTS ( 'NONE', 3,
 ( #10855, #18536, #28723, #20690, #16243, #28570, #26420, #3611, #3450, #18858, #30874, #1145, #26263, #16404, #31037, #3288, #30716, #3943, #11014, #28895, #8226, #989, #13635, #23641, #21159, #10703, #3772, #28411, #673, #13795, #21003, #11330, #23154, #15926 ),
 .UNSPECIFIED., .F., .F.,
 ( 4, 2, 2, 2, 2, 2, 2, 2, 2, 2, 2, 2, 2, 2, 2, 2, 4 ),
 ( 0.000000000000000000, 0.03125000000000000694, 0.06250000000000001388, 0.09375000000000002776, 0.1250000000000000278, 0.1562500000000000278, 0.1875000000000000555, 0.2187500000000000278, 0.2500000000000000000, 0.2812500000000000000, 0.3125000000000000000, 0.3437500000000000000, 0.3750000000000000000, 0.4062500000000000555, 0.4375000000000000555, 0.4687500000000000555, 0.5000000000000000000 ),
 .UNSPECIFIED. ) ;
#26414=ORIENTED_EDGE ( 'NONE', *, *, #18477, .F. ) ;
#26417=CARTESIAN_POINT ( 'NONE',  ( 21.09785597605720042, -13.88867167006704939, 47.04930799450051637 ) ) ;
#26420=CARTESIAN_POINT ( 'NONE',  ( -6.872792942851614129, -13.30632128221581212, -1.386849490760369008 ) ) ;
#26421=EDGE_CURVE ( 'NONE', #1958, #9202, #3065, .T. ) ;
#26430=DIRECTION ( 'NONE',  ( 0.000000000000000000, 0.000000000000000000, 1.000000000000000000 ) ) ;
#26435=EDGE_LOOP ( 'NONE', ( #25836, #16728, #26906, #18981 ) ) ;
#26439=VERTEX_POINT ( 'NONE', #9367 ) ;
#26454=ORIENTED_EDGE ( 'NONE', *, *, #11379, .T. ) ;
#26467=AXIS2_PLACEMENT_3D ( 'NONE', #2610, #22305, #22457 ) ;
#26505=CARTESIAN_POINT ( 'NONE',  ( 21.09785597605720753, -13.59284023713420630, 102.7732403313682994 ) ) ;
#26512=CARTESIAN_POINT ( 'NONE',  ( 21.09785597605720753, -13.59284023713420630, 102.6732403313682909 ) ) ;
#26529=EDGE_CURVE ( 'NONE', #756, #12577, #2515, .T. ) ;
#26532=EDGE_LOOP ( 'NONE', ( #15102, #1528, #29060, #5297 ) ) ;
#26538=PRODUCT_DEFINITION_FORMATION_WITH_SPECIFIED_SOURCE ( 'ANY', '', #20053, .NOT_KNOWN. ) ;
#26554=FACE_OUTER_BOUND ( 'NONE', #20225, .T. ) ;
#26556=DIRECTION ( 'NONE',  ( 0.000000000000000000, 0.000000000000000000, -1.000000000000000000 ) ) ;
#26558=ORIENTED_EDGE ( 'NONE', *, *, #12061, .T. ) ;
#26597=ORIENTED_EDGE ( 'NONE', *, *, #7159, .T. ) ;
#26623=CARTESIAN_POINT ( 'NONE',  ( 17.28711060612849337, -13.74047052604243824, -11.17459240441506019 ) ) ;
#26649=ORIENTED_EDGE ( 'NONE', *, *, #329, .F. ) ;
#26651=ORIENTED_EDGE ( 'NONE', *, *, #14390, .T. ) ;
#26667=EDGE_CURVE ( 'NONE', #18606, #21751, #28766, .T. ) ;
#26693=CARTESIAN_POINT ( 'NONE',  ( 21.09785597605719332, 7.881678200673687407, 27.79103836896735302 ) ) ;
#26708=VERTEX_POINT ( 'NONE', #9658 ) ;
#26755=CARTESIAN_POINT ( 'NONE',  ( 21.09785597605720042, -17.03545420775220265, -31.35069200549948221 ) ) ;
#26760=CARTESIAN_POINT ( 'NONE',  ( 69.53401346131808225, -13.30632128221581212, 19.07865907559169472 ) ) ;
#26767=CARTESIAN_POINT ( 'NONE',  ( 73.43141673955737758, -13.74047052604243646, 72.85129969572992081 ) ) ;
#26787=CIRCLE ( 'NONE', #24690, 55.96105416618080142 ) ;
#26789=DIRECTION ( 'NONE',  ( -0.000000000000000000, -1.000000000000000000, -0.000000000000000000 ) ) ;
#26813=DIRECTION ( 'NONE',  ( 0.000000000000000000, 1.000000000000000000, 0.000000000000000000 ) ) ;
#26822=ADVANCED_FACE ( 'NONE', ( #9498 ), #14551, .F. ) ;
#26906=ORIENTED_EDGE ( 'NONE', *, *, #18618, .T. ) ;
#26907=DIRECTION ( 'NONE',  ( 0.000000000000000000, 1.000000000000000000, -0.000000000000000000 ) ) ;
#26915=ORIENTED_EDGE ( 'NONE', *, *, #5037, .F. ) ;
#26951=CARTESIAN_POINT ( 'NONE',  ( -29.43068460852080293, -13.74047052604243646, 76.22825493111784567 ) ) ;
#26959=TOROIDAL_SURFACE ( 'NONE', #2853, 13.98419020052803852, 1.000000000001014744 ) ;
#26988=AXIS2_PLACEMENT_3D ( 'NONE', #15776, #22993, #5449 ) ;
#26990=AXIS2_PLACEMENT_3D ( 'NONE', #10369, #13644, #23160 ) ;
#26992=VERTEX_POINT ( 'NONE', #10432 ) ;
#27013=AXIS2_PLACEMENT_3D ( 'NONE', #30519, #23437, #12800 ) ;
#27034=ORIENTED_EDGE ( 'NONE', *, *, #16802, .F. ) ;
#27041=DIRECTION ( 'NONE',  ( 0.000000000000000000, 0.000000000000000000, -1.000000000000000000 ) ) ;
#27075=CARTESIAN_POINT ( 'NONE',  ( 21.09785597605720042, -13.59284023713420630, -8.674624342367264873 ) ) ;
#27082=CIRCLE ( 'NONE', #17120, 12.78419020052701960 ) ;
#27084=ADVANCED_FACE ( 'NONE', ( #6627 ), #4698, .T. ) ;
#27099=CARTESIAN_POINT ( 'NONE',  ( 21.09785597605719332, 7.264443105416139801, 47.04930799450051637 ) ) ;
#27104=CARTESIAN_POINT ( 'NONE',  ( 21.09785597605719332, 15.43591091851532759, 61.03349819502855667 ) ) ;
#27113=CARTESIAN_POINT ( 'NONE',  ( -37.12604442285837081, -13.74047052604243646, 50.86005336442920566 ) ) ;
#27142=VERTEX_POINT ( 'NONE', #16618 ) ;
#27147=ORIENTED_EDGE ( 'NONE', *, *, #17151, .F. ) ;
#27150=CARTESIAN_POINT ( 'NONE',  ( 21.09785597605720042, -14.03534765547855656, 47.04930799450051637 ) ) ;
#27175=TOROIDAL_SURFACE ( 'NONE', #8297, 70.59901951359279337, 1.000000000000000444 ) ;
#27179=ORIENTED_EDGE ( 'NONE', *, *, #14847, .F. ) ;
#27193=CARTESIAN_POINT ( 'NONE',  ( 21.09785597605720042, -14.04221034894631615, 47.04930799450051637 ) ) ;
#27203=CARTESIAN_POINT ( 'NONE',  ( 21.09785597605719332, 17.16451738380053271, 47.04930799450051637 ) ) ;
#27208=EDGE_LOOP ( 'NONE', ( #32388, #10016, #13820, #27555 ) ) ;
#27213=CARTESIAN_POINT ( 'NONE',  ( 21.09785597605721463, -16.93545420775220123, 125.5493079945005093 ) ) ;
#27248=ORIENTED_EDGE ( 'NONE', *, *, #6774, .T. ) ;
#27277=CARTESIAN_POINT ( 'NONE',  ( -37.12604442285837791, -13.74047052604243646, 43.23856262457184840 ) ) ;
#27338=CARTESIAN_POINT ( 'NONE',  ( 21.09785597605720042, -16.03545420775220265, 47.04930799450051637 ) ) ;
#27345=AXIS2_PLACEMENT_3D ( 'NONE', #25234, #2745, #20458 ) ;
#27372=AXIS2_PLACEMENT_3D ( 'NONE', #16012, #26789, #19719 ) ;
#27393=EDGE_CURVE ( 'NONE', #11333, #22659, #10234, .T. ) ;
#27414=ORIENTED_EDGE ( 'NONE', *, *, #10409, .F. ) ;
#27418=DIRECTION ( 'NONE',  ( 0.000000000000000000, 0.000000000000000000, -1.000000000000000000 ) ) ;
#27429=CIRCLE ( 'NONE', #7521, 0.1999999999999987899 ) ;
#27453=( NAMED_UNIT ( * ) PLANE_ANGLE_UNIT ( ) SI_UNIT ( $, .RADIAN. ) );
#27469=ADVANCED_FACE ( 'NONE', ( #15154 ), #16775, .F. ) ;
#27491=CARTESIAN_POINT ( 'NONE',  ( 21.09785597605720042, -13.37218737171702543, -8.638398481670979123 ) ) ;
#27497=ADVANCED_FACE ( 'NONE', ( #11351 ), #21479, .T. ) ;
#27501=DIRECTION ( 'NONE',  ( 0.000000000000000000, 0.000000000000000000, -1.000000000000000000 ) ) ;
#27515=TOROIDAL_SURFACE ( 'NONE', #3918, 12.78419020052701960, 0.2000000000000000944 ) ;
#27524=VERTEX_POINT ( 'NONE', #13982 ) ;
#27537=CIRCLE ( 'NONE', #26467, 59.44168675549763492 ) ;
#27544=CIRCLE ( 'NONE', #11281, 70.59901951359279337 ) ;
#27547=ADVANCED_FACE ( 'NONE', ( #1168 ), #3147, .F. ) ;
#27555=ORIENTED_EDGE ( 'NONE', *, *, #31935, .T. ) ;
#27562=DIRECTION ( 'NONE',  ( 0.000000000000000000, 0.000000000000000000, -1.000000000000000000 ) ) ;
#27644=AXIS2_PLACEMENT_3D ( 'NONE', #3802, #24147, #7083 ) ;
#27659=EDGE_CURVE ( 'NONE', #27524, #27708, #15762, .T. ) ;
#27667=ORIENTED_EDGE ( 'NONE', *, *, #16802, .T. ) ;
#27679=ADVANCED_FACE ( 'NONE', ( #32354 ), #2595, .F. ) ;
#27707=VECTOR ( 'NONE', #24055, 1000.000000000000000 ) ;
#27708=VERTEX_POINT ( 'NONE', #31700 ) ;
#27712=ADVANCED_FACE ( 'NONE', ( #9545 ), #18883, .F. ) ;
#27721=TOROIDAL_SURFACE ( 'NONE', #24027, 55.78321279447762748, 0.1000000000000016986 ) ;
#27733=DIRECTION ( 'NONE',  ( -1.000000000000000000, 0.000000000000000000, 0.000000000000000000 ) ) ;
#27749=CARTESIAN_POINT ( 'NONE',  ( 21.09785597605720042, -16.03545420775220265, -23.54971151909227700 ) ) ;
#27769=DIRECTION ( 'NONE',  ( 0.000000000000000000, -1.000000000000000000, 0.000000000000000000 ) ) ;
#27781=ORIENTED_EDGE ( 'NONE', *, *, #15872, .F. ) ;
#27794=AXIS2_PLACEMENT_3D ( 'NONE', #6450, #19064, #29093 ) ;
#27826=DIRECTION ( 'NONE',  ( 0.000000000000000000, 1.000000000000000000, -0.000000000000000000 ) ) ;
#27831=AXIS2_PLACEMENT_3D ( 'NONE', #22068, #6981, #24215 ) ;
#27839=CIRCLE ( 'NONE', #23631, 0.1999999999999918510 ) ;
#27856=FACE_OUTER_BOUND ( 'NONE', #18850, .T. ) ;
#27915=TOROIDAL_SURFACE ( 'NONE', #21077, 83.95481021798164534, 94.94530576803616384 ) ;
#27918=AXIS2_PLACEMENT_3D ( 'NONE', #18012, #4899, #5222 ) ;
#27949=VERTEX_POINT ( 'NONE', #28232 ) ;
#27986=ORIENTED_EDGE ( 'NONE', *, *, #32402, .T. ) ;
#27996=ADVANCED_FACE ( 'NONE', ( #18841 ), #24142, .T. ) ;
#28071=EDGE_LOOP ( 'NONE', ( #5477, #29528, #4668, #19627 ) ) ;
#28077=AXIS2_PLACEMENT_3D ( 'NONE', #29010, #16522, #14077 ) ;
#28101=CYLINDRICAL_SURFACE ( 'NONE', #2158, 12.98419020052702599 ) ;
#28105=( NAMED_UNIT ( * ) SI_UNIT ( $, .STERADIAN. ) SOLID_ANGLE_UNIT ( ) );
#28141=DIRECTION ( 'NONE',  ( -0.000000000000000000, -1.000000000000000000, -0.000000000000000000 ) ) ;
#28163=DIRECTION ( 'NONE',  ( 0.000000000000000000, 0.000000000000000000, -1.000000000000000000 ) ) ;
#28177=VERTEX_POINT ( 'NONE', #27213 ) ;
#28182=DIRECTION ( 'NONE',  ( 0.000000000000000000, 1.000000000000000000, -0.000000000000000000 ) ) ;
#28189=DIRECTION ( 'NONE',  ( 0.000000000000000000, 0.000000000000000000, -1.000000000000000000 ) ) ;
#28228=CIRCLE ( 'NONE', #3042, 0.1000000000000028644 ) ;
#28232=CARTESIAN_POINT ( 'NONE',  ( 21.09785597605719332, 15.43591091851533115, 60.03349819502753348 ) ) ;
#28259=ORIENTED_EDGE ( 'NONE', *, *, #26421, .F. ) ;
#28294=CARTESIAN_POINT ( 'NONE',  ( 21.09785597605720042, -13.88867167006704939, 47.04930799450051637 ) ) ;
#28299=ORIENTED_EDGE ( 'NONE', *, *, #15168, .T. ) ;
#28304=DIRECTION ( 'NONE',  ( 1.000000000000000000, 0.000000000000000000, -1.224646799147353207E-16 ) ) ;
#28312=CARTESIAN_POINT ( 'NONE',  ( 21.09785597605718976, 6.717634499306958773, 67.32574359352868498 ) ) ;
#28350=( LENGTH_UNIT ( ) NAMED_UNIT ( * ) SI_UNIT ( .MILLI., .METRE. ) );
#28403=CIRCLE ( 'NONE', #7955, 0.1000000000000028644 ) ;
#28411=CARTESIAN_POINT ( 'NONE',  ( -6.872792942851601694, -13.30632128221581034, 95.48546547976137333 ) ) ;
#28421=CARTESIAN_POINT ( 'NONE',  ( 21.09785597605719332, -13.49020584019834601, 47.04930799450051637 ) ) ;
#28427=CARTESIAN_POINT ( 'NONE',  ( 39.08163115802605603, -13.30632128221581212, 100.0115811999271358 ) ) ;
#28437=TOROIDAL_SURFACE ( 'NONE', #16888, 64.50000000000000000, 5.499019513592785735 ) ;
#28442=CIRCLE ( 'NONE', #730, 0.09999999999998898659 ) ;
#28450=DIRECTION ( 'NONE',  ( 0.000000000000000000, 1.000000000000000000, -0.000000000000000000 ) ) ;
#28469=DIRECTION ( 'NONE',  ( 0.000000000000000000, 0.000000000000000000, -1.000000000000000000 ) ) ;
#28470=CARTESIAN_POINT ( 'NONE',  ( 21.09785597605720753, -14.54791319078308653, 105.5132833334411515 ) ) ;
#28472=EDGE_LOOP ( 'NONE', ( #13534, #10611, #25497, #24794 ) ) ;
#28493=AXIS2_PLACEMENT_3D ( 'NONE', #3385, #10795, #20944 ) ;
#28510=CIRCLE ( 'NONE', #2816, 19.25826962553310295 ) ;
#28535=ORIENTED_EDGE ( 'NONE', *, *, #7159, .F. ) ;
#28547=TOROIDAL_SURFACE ( 'NONE', #3366, 58.86319174311611846, 0.1999999999999984290 ) ;
#28557=ORIENTED_EDGE ( 'NONE', *, *, #24855, .T. ) ;
#28570=CARTESIAN_POINT ( 'NONE',  ( -3.635677172050070460, -13.30632128221581567, -3.117123918615727352 ) ) ;
#28609=EDGE_CURVE ( 'NONE', #15162, #15932, #12613, .T. ) ;
#28615=DIRECTION ( 'NONE',  ( -0.000000000000000000, -1.000000000000000000, -0.000000000000000000 ) ) ;
#28638=CIRCLE ( 'NONE', #1904, 78.39999999999999147 ) ;
#28652=DIRECTION ( 'NONE',  ( 1.000000000000000000, 0.000000000000000000, -1.224646799147353207E-16 ) ) ;
#28679=VERTEX_POINT ( 'NONE', #30239 ) ;
#28693=DIRECTION ( 'NONE',  ( 0.000000000000000000, 0.000000000000000000, -1.000000000000000000 ) ) ;
#28711=CIRCLE ( 'NONE', #5118, 36.51080762834750715 ) ;
#28723=CARTESIAN_POINT ( 'NONE',  ( 13.79206092585403454, -13.30632128221581212, -8.403770473392276230 ) ) ;
#28740=EDGE_LOOP ( 'NONE', ( #27179, #20088, #6191, #30431 ) ) ;
#28759=ORIENTED_EDGE ( 'NONE', *, *, #6523, .F. ) ;
#28766=CIRCLE ( 'NONE', #5649, 19.21451602543517367 ) ;
#28768=DIRECTION ( 'NONE',  ( 0.000000000000000000, 0.000000000000000000, -1.000000000000000000 ) ) ;
#28785=CARTESIAN_POINT ( 'NONE',  ( 21.09785597605719332, 17.16451738380053627, 34.36516646732340519 ) ) ;
#28801=CIRCLE ( 'NONE', #10477, 0.5999999999999980904 ) ;
#28811=DIRECTION ( 'NONE',  ( 0.000000000000000000, 0.000000000000000000, -1.000000000000000000 ) ) ;
#28851=FACE_OUTER_BOUND ( 'NONE', #4911, .T. ) ;
#28881=DIRECTION ( 'NONE',  ( -0.000000000000000000, -1.000000000000000000, -0.000000000000000000 ) ) ;
#28887=TOROIDAL_SURFACE ( 'NONE', #14731, 64.50000000000000000, 5.499019513592785735 ) ;
#28895=CARTESIAN_POINT ( 'NONE',  ( -32.92991496113891259, -13.30632128221581212, 61.52060788219944953 ) ) ;
#28918=CARTESIAN_POINT ( 'NONE',  ( 79.32175637497276455, -13.74047052604243646, 43.23856262457181998 ) ) ;
#28922=TOROIDAL_SURFACE ( 'NONE', #14767, 12.68414152717710763, 0.1999999999999992339 ) ;
#28957=DIRECTION ( 'NONE',  ( -1.000000000000000000, 0.000000000000000000, 0.000000000000000000 ) ) ;
#28961=SPHERICAL_SURFACE ( 'NONE', #3602, 36.01080762834750715 ) ;
#28969=ORIENTED_EDGE ( 'NONE', *, *, #10287, .T. ) ;
#28988=EDGE_CURVE ( 'NONE', #18054, #10039, #12630, .T. ) ;
#29010=CARTESIAN_POINT ( 'NONE',  ( 21.09785597605718266, 77.37245976740706510, 131.0041182124821830 ) ) ;
#29024=CARTESIAN_POINT ( 'NONE',  ( 21.09785597605719332, 77.37245976740706510, 47.04930799450051637 ) ) ;
#29038=DIRECTION ( 'NONE',  ( 0.000000000000000000, 1.000000000000000000, 0.000000000000000000 ) ) ;
#29040=ORIENTED_EDGE ( 'NONE', *, *, #21571, .T. ) ;
#29052=VERTEX_POINT ( 'NONE', #24951 ) ;
#29060=ORIENTED_EDGE ( 'NONE', *, *, #17792, .T. ) ;
#29066=CARTESIAN_POINT ( 'NONE',  ( 78.94643999631821885, -13.74047052604243113, 39.42791148283190239 ) ) ;
#29087=DIRECTION ( 'NONE',  ( 0.000000000000000000, 0.000000000000000000, -1.000000000000000000 ) ) ;
#29092=CARTESIAN_POINT ( 'NONE',  ( -34.15232302351033411, -13.74047052604243646, 28.28865559504964011 ) ) ;
#29093=DIRECTION ( 'NONE',  ( 0.000000000000000000, 0.000000000000000000, -1.000000000000000000 ) ) ;
#29096=CIRCLE ( 'NONE', #23867, 0.09999999999999766020 ) ;
#29124=CARTESIAN_POINT ( 'NONE',  ( 21.09785597605719332, 7.264443105416139801, 27.83479196906534625 ) ) ;
#29129=DIRECTION ( 'NONE',  ( 0.000000000000000000, 0.000000000000000000, -1.000000000000000000 ) ) ;
#29143=CARTESIAN_POINT ( 'NONE',  ( 21.09785597605720042, -16.03545420775219910, 47.04930799450051637 ) ) ;
#29149=CARTESIAN_POINT ( 'NONE',  ( 21.09785597605719332, 15.43591091851533115, 34.06511779397349926 ) ) ;
#29166=CARTESIAN_POINT ( 'NONE',  ( 21.09785597605718976, 7.881678200673687407, 66.30757762003366906 ) ) ;
#29168=DIRECTION ( 'NONE',  ( 0.000000000000000000, 0.000000000000000000, -1.000000000000000000 ) ) ;
#29211=CARTESIAN_POINT ( 'NONE',  ( 21.09785597605719332, 77.37245976740706510, 47.04930799450051637 ) ) ;
#29228=CARTESIAN_POINT ( 'NONE',  ( 77.45956091363653684, -13.74047052604244001, 31.95286555045028720 ) ) ;
#29230=DIRECTION ( 'NONE',  ( 0.000000000000000000, 0.000000000000000000, -1.000000000000000000 ) ) ;
#29234=CARTESIAN_POINT ( 'NONE',  ( 21.09785597605720753, -14.04221034894631615, 105.9124997376166277 ) ) ;
#29248=CARTESIAN_POINT ( 'NONE',  ( 2.337203576606338373, -13.74047052604243646, 102.2994869940680474 ) ) ;
#29318=AXIS2_PLACEMENT_3D ( 'NONE', #1658, #11681, #19369 ) ;
#29328=ADVANCED_FACE ( 'NONE', ( #8998 ), #14726, .T. ) ;
#29336=DIRECTION ( 'NONE',  ( 0.000000000000000000, 0.000000000000000000, -1.000000000000000000 ) ) ;
#29355=ORIENTED_EDGE ( 'NONE', *, *, #6257, .T. ) ;
#29401=CARTESIAN_POINT ( 'NONE',  ( 21.09785597605720042, -16.03545420775219910, 47.04930799450051637 ) ) ;
#29462=ORIENTED_EDGE ( 'NONE', *, *, #21807, .F. ) ;
#29482=CIRCLE ( 'NONE', #1674, 94.94530576803560962 ) ;
#29507=ORIENTED_EDGE ( 'NONE', *, *, #26257, .T. ) ;
#29512=DIRECTION ( 'NONE',  ( 0.000000000000000000, 0.000000000000000000, -1.000000000000000000 ) ) ;
#29528=ORIENTED_EDGE ( 'NONE', *, *, #17151, .T. ) ;
#29533=EDGE_CURVE ( 'NONE', #11078, #6225, #29943, .T. ) ;
#29534=EDGE_CURVE ( 'NONE', #3864, #6225, #23138, .T. ) ;
#29566=CARTESIAN_POINT ( 'NONE',  ( 46.89984767728661552, -13.74047052604243646, 99.38286875800068287 ) ) ;
#29570=DIRECTION ( 'NONE',  ( 0.000000000000000000, 0.000000000000000000, -1.000000000000000000 ) ) ;
#29586=CARTESIAN_POINT ( 'NONE',  ( -8.081090960560100456, -13.74047052604243646, 97.57784857907851972 ) ) ;
#29601=VERTEX_POINT ( 'NONE', #23095 ) ;
#29605=CIRCLE ( 'NONE', #11796, 0.1999999999999918510 ) ;
#29611=ORIENTED_EDGE ( 'NONE', *, *, #30755, .T. ) ;
#29612=ORIENTED_EDGE ( 'NONE', *, *, #1166, .T. ) ;
#29637=DIRECTION ( 'NONE',  ( 0.000000000000000000, 1.000000000000000000, -0.000000000000000000 ) ) ;
#29666=VERTEX_POINT ( 'NONE', #29149 ) ;
#29693=EDGE_CURVE ( 'NONE', #14944, #28177, #6986, .T. ) ;
#29716=ORIENTED_EDGE ( 'NONE', *, *, #11094, .T. ) ;
#29724=CARTESIAN_POINT ( 'NONE',  ( 21.09785597605718266, 77.37245976740706510, 131.0041182124821830 ) ) ;
#29726=ORIENTED_EDGE ( 'NONE', *, *, #14390, .F. ) ;
#29729=ADVANCED_FACE ( 'NONE', ( #6503 ), #7943, .F. ) ;
#29736=AXIS2_PLACEMENT_3D ( 'NONE', #8603, #8916, #28469 ) ;
#29747=CARTESIAN_POINT ( 'NONE',  ( -34.15232302351031279, -13.74047052604243646, 65.80996039395141395 ) ) ;
#29776=CARTESIAN_POINT ( 'NONE',  ( 21.09785597605719332, 34.11266481626051217, 34.56516646732339382 ) ) ;
#29792=ORIENTED_EDGE ( 'NONE', *, *, #5943, .T. ) ;
#29804=CARTESIAN_POINT ( 'NONE',  ( 21.09785597605719332, 34.11266481626051217, 47.04930799450051637 ) ) ;
#29814=AXIS2_PLACEMENT_3D ( 'NONE', #6402, #11175, #31198 ) ;
#29826=SPHERICAL_SURFACE ( 'NONE', #6000, 36.51080762834750715 ) ;
#29828=DIRECTION ( 'NONE',  ( 0.000000000000000000, 0.000000000000000000, -1.000000000000000000 ) ) ;
#29836=CARTESIAN_POINT ( 'NONE',  ( 21.09785597605719332, 15.24673779880127356, 33.56516646732238485 ) ) ;
#29857=ADVANCED_FACE ( 'NONE', ( #4683 ), #29969, .T. ) ;
#29860=CIRCLE ( 'NONE', #11000, 5.099019513592786268 ) ;
#29863=FACE_OUTER_BOUND ( 'NONE', #5248, .T. ) ;
#29876=VERTEX_POINT ( 'NONE', #28470 ) ;
#29878=CARTESIAN_POINT ( 'NONE',  ( 21.09785597605719332, 6.671061906060458568, 47.04930799450051637 ) ) ;
#29891=EDGE_LOOP ( 'NONE', ( #19527, #29716, #6743, #5409 ) ) ;
#29897=DIRECTION ( 'NONE',  ( 0.000000000000000000, 0.000000000000000000, 1.000000000000000000 ) ) ;
#29914=CIRCLE ( 'NONE', #11052, 58.46397533894063514 ) ;
#29917=FACE_OUTER_BOUND ( 'NONE', #23008, .T. ) ;
#29923=SURFACE_STYLE_USAGE ( .BOTH. , #32376 ) ;
#29932=CARTESIAN_POINT ( 'NONE',  ( 21.09785597605719332, 6.547041198165487685, 26.66847926540308933 ) ) ;
#29943=CIRCLE ( 'NONE', #5840, 69.99901951359278485 ) ;
#29968=ORIENTED_EDGE ( 'NONE', *, *, #14617, .F. ) ;
#29969=TOROIDAL_SURFACE ( 'NONE', #15805, 20.27643559902816861, 0.2000000000000001499 ) ;
#29974=DIRECTION ( 'NONE',  ( -0.000000000000000000, -1.000000000000000000, -0.000000000000000000 ) ) ;
#30037=VERTEX_POINT ( 'NONE', #6297 ) ;
#30046=PRODUCT_CONTEXT ( 'NONE', #17040, 'mechanical' ) ;
#30060=CONICAL_SURFACE ( 'NONE', #20603, 58.67217910650386159, 0.3009234521321452749 ) ;
#30070=TOROIDAL_SURFACE ( 'NONE', #28493, 78.39999999999999147, 0.1000000000000014211 ) ;
#30082=CARTESIAN_POINT ( 'NONE',  ( 21.09785597605720753, -16.63545420775220407, 117.6483275080933169 ) ) ;
#30088=ORIENTED_EDGE ( 'NONE', *, *, #31710, .F. ) ;
#30137=CARTESIAN_POINT ( 'NONE',  ( 21.09785597605719332, 17.16451738380053271, 34.06511779397349216 ) ) ;
#30139=FACE_OUTER_BOUND ( 'NONE', #14342, .T. ) ;
#30140=EDGE_LOOP ( 'NONE', ( #17737, #32273, #5978, #1683 ) ) ;
#30169=DIRECTION ( 'NONE',  ( 0.000000000000000000, 1.000000000000000000, -0.000000000000000000 ) ) ;
#30184=VERTEX_POINT ( 'NONE', #4485 ) ;
#30185=EDGE_CURVE ( 'NONE', #5958, #11143, #18439, .T. ) ;
#30189=ORIENTED_EDGE ( 'NONE', *, *, #15263, .F. ) ;
#30195=ORIENTED_EDGE ( 'NONE', *, *, #31517, .F. ) ;
#30201=CARTESIAN_POINT ( 'NONE',  ( 21.09785597605720753, -16.03545420775219910, 111.5493079945005235 ) ) ;
#30218=EDGE_CURVE ( 'NONE', #9202, #1958, #3773, .T. ) ;
#30239=CARTESIAN_POINT ( 'NONE',  ( 21.09785597605718621, -12.82881809906321813, -8.911746171680242412 ) ) ;
#30241=FILL_AREA_STYLE_COLOUR ( '', #5031 ) ;
#30256=DIRECTION ( 'NONE',  ( 0.000000000000000000, 1.000000000000000000, -0.000000000000000000 ) ) ;
#30289=CIRCLE ( 'NONE', #14552, 1.000000000001013856 ) ;
#30306=CARTESIAN_POINT ( 'NONE',  ( 21.09785597605720042, -13.56320000832927875, 47.04930799450051637 ) ) ;
#30318=DIRECTION ( 'NONE',  ( -0.000000000000000000, -1.000000000000000000, -0.000000000000000000 ) ) ;
#30326=EDGE_CURVE ( 'NONE', #22362, #26708, #26334, .T. ) ;
#30347=CONICAL_SURFACE ( 'NONE', #21937, 58.67217910650386159, 0.3009234521321452749 ) ;
#30388=DIRECTION ( 'NONE',  ( -1.000000000000000000, 0.000000000000000000, -1.224646799147353207E-16 ) ) ;
#30431=ORIENTED_EDGE ( 'NONE', *, *, #13674, .F. ) ;
#30480=CARTESIAN_POINT ( 'NONE',  ( 21.09785597605720042, -17.03545420775220265, -23.54971151909227700 ) ) ;
#30483=AXIS2_PLACEMENT_3D ( 'NONE', #16292, #26143, #31725 ) ;
#30492=FACE_OUTER_BOUND ( 'NONE', #13539, .T. ) ;
#30502=FACE_OUTER_BOUND ( 'NONE', #28472, .T. ) ;
#30513=ADVANCED_FACE ( 'NONE', ( #12622 ), #16353, .T. ) ;
#30519=CARTESIAN_POINT ( 'NONE',  ( 21.09785597605719332, -13.49020584019834601, 47.04930799450051637 ) ) ;
#30534=ORIENTED_EDGE ( 'NONE', *, *, #2683, .F. ) ;
#30559=CARTESIAN_POINT ( 'NONE',  ( 21.09785597605720042, -13.56320000832927875, 47.04930799450051637 ) ) ;
#30569=AXIS2_PLACEMENT_3D ( 'NONE', #6525, #1590, #11613 ) ;
#30573=CARTESIAN_POINT ( 'NONE',  ( 45.83138912416445265, -13.30632128221581389, 97.21573990761677919 ) ) ;
#30584=DIRECTION ( 'NONE',  ( 0.000000000000000000, 0.000000000000000000, -1.000000000000000000 ) ) ;
#30590=AXIS2_PLACEMENT_3D ( 'NONE', #16502, #21582, #21745 ) ;
#30628=ADVANCED_FACE ( 'NONE', ( #30502 ), #5062, .T. ) ;
#30658=DIRECTION ( 'NONE',  ( -0.000000000000000000, -1.000000000000000000, -0.000000000000000000 ) ) ;
#30662=ORIENTED_EDGE ( 'NONE', *, *, #10231, .F. ) ;
#30672=DIRECTION ( 'NONE',  ( 0.000000000000000000, 0.000000000000000000, -1.000000000000000000 ) ) ;
#30674=VECTOR ( 'NONE', #2774, 1000.000000000000000 ) ;
#30688=DIRECTION ( 'NONE',  ( -0.000000000000000000, -1.000000000000000000, -0.000000000000000000 ) ) ;
#30716=CARTESIAN_POINT ( 'NONE',  ( -34.71499704722535284, -13.30632128221581212, 43.39636530629570643 ) ) ;
#30718=FACE_BOUND ( 'NONE', #11157, .T. ) ;
#30735=DIRECTION ( 'NONE',  ( 0.000000000000000000, 1.000000000000000000, -0.000000000000000000 ) ) ;
#30755=EDGE_CURVE ( 'NONE', #23707, #30037, #9053, .T. ) ;
#30802=FACE_OUTER_BOUND ( 'NONE', #17385, .T. ) ;
#30818=DIRECTION ( 'NONE',  ( 1.000000000000000000, 0.000000000000000000, -1.224646799147353207E-16 ) ) ;
#30842=ORIENTED_EDGE ( 'NONE', *, *, #30218, .F. ) ;
#30843=CARTESIAN_POINT ( 'NONE',  ( 21.09785597605720042, -14.04221034894631615, 47.04930799450051637 ) ) ;
#30861=CIRCLE ( 'NONE', #29814, 0.2000000000000022593 ) ;
#30863=AXIS2_PLACEMENT_3D ( 'NONE', #31186, #1455, #10998 ) ;
#30874=CARTESIAN_POINT ( 'NONE',  ( -23.27936906821728869, -13.30632128221581212, 13.00403739414156590 ) ) ;
#30892=AXIS2_PLACEMENT_3D ( 'NONE', #12751, #20914, #18132 ) ;
#30915=CARTESIAN_POINT ( 'NONE',  ( 21.09785597605720753, -14.24176827912842391, 105.8992094215394388 ) ) ;
#30920=DIRECTION ( 'NONE',  ( 0.000000000000000000, 0.000000000000000000, -1.000000000000000000 ) ) ;
#30921=CARTESIAN_POINT ( 'NONE',  ( 21.09785597605720042, -16.93545420775220123, 47.04930799450051637 ) ) ;
#30940=DIRECTION ( 'NONE',  ( 0.000000000000000000, 0.000000000000000000, 1.000000000000000000 ) ) ;
#30944=EDGE_LOOP ( 'NONE', ( #5991, #17160, #12766, #18020, #22159 ) ) ;
#30950=AXIS2_PLACEMENT_3D ( 'NONE', #28294, #23364, #30920 ) ;
#30976=ORIENTED_EDGE ( 'NONE', *, *, #31710, .T. ) ;
#30989=ORIENTED_EDGE ( 'NONE', *, *, #10097, .T. ) ;
#30990=EDGE_CURVE ( 'NONE', #26992, #11078, #664, .T. ) ;
#30992=ADVANCED_FACE ( 'NONE', ( #30139 ), #10120, .T. ) ;
#31007=DIRECTION ( 'NONE',  ( 0.000000000000000000, 0.000000000000000000, -1.000000000000000000 ) ) ;
#31025=CIRCLE ( 'NONE', #6913, 1.000000000001013856 ) ;
#31037=CARTESIAN_POINT ( 'NONE',  ( -32.92991496113891259, -13.30632128221581567, 32.57800810680159742 ) ) ;
#31043=ORIENTED_EDGE ( 'NONE', *, *, #6481, .F. ) ;
#31055=ORIENTED_EDGE ( 'NONE', *, *, #24979, .T. ) ;
#31099=DIRECTION ( 'NONE',  ( 0.000000000000000000, 0.000000000000000000, 1.000000000000000000 ) ) ;
#31135=FACE_OUTER_BOUND ( 'NONE', #19689, .T. ) ;
#31146=VERTEX_POINT ( 'NONE', #20595 ) ;
#31176=CIRCLE ( 'NONE', #15980, 0.6000000000000033085 ) ;
#31186=CARTESIAN_POINT ( 'NONE',  ( 21.09785597605719332, 7.264443105416139801, 47.04930799450051637 ) ) ;
#31196=AXIS2_PLACEMENT_3D ( 'NONE', #4259, #26907, #31516 ) ;
#31198=DIRECTION ( 'NONE',  ( 0.000000000000000000, 0.000000000000000000, -1.000000000000000000 ) ) ;
#31207=EDGE_LOOP ( 'NONE', ( #17373, #18818, #1846, #20158 ) ) ;
#31209=CARTESIAN_POINT ( 'NONE',  ( 28.40365102626035565, -13.30632128221581034, 102.5023864623932894 ) ) ;
#31221=EDGE_LOOP ( 'NONE', ( #3455, #26558, #6792, #8293 ) ) ;
#31222=CARTESIAN_POINT ( 'NONE',  ( 21.09785597605720042, -16.93545420775220478, 47.04930799450051637 ) ) ;
#31224=ADVANCED_FACE ( 'NONE', ( #9586 ), #30060, .T. ) ;
#31237=EDGE_CURVE ( 'NONE', #24256, #6225, #7520, .T. ) ;
#31262=ORIENTED_EDGE ( 'NONE', *, *, #26421, .T. ) ;
#31350=DIRECTION ( 'NONE',  ( 0.000000000000000000, 0.000000000000000000, -1.000000000000000000 ) ) ;
#31374=EDGE_LOOP ( 'NONE', ( #18930, #31055, #16852, #29726 ) ) ;
#31402=CARTESIAN_POINT ( 'NONE',  ( 21.09785597605720753, -14.03534765547855656, 106.8589376701495581 ) ) ;
#31411=EDGE_LOOP ( 'NONE', ( #23120, #13592, #30195, #4657 ) ) ;
#31421=ORIENTED_EDGE ( 'NONE', *, *, #30990, .T. ) ;
#31473=CARTESIAN_POINT ( 'NONE',  ( 21.09785597605720042, -52.14605111273580462, 47.04930799450051637 ) ) ;
#31488=PLANE ( 'NONE',  #1181 ) ;
#31494=CARTESIAN_POINT ( 'NONE',  ( 21.09785597605719332, 17.36451738380053555, 47.04930799450051637 ) ) ;
#31516=DIRECTION ( 'NONE',  ( 0.000000000000000000, 0.000000000000000000, -1.000000000000000000 ) ) ;
#31517=EDGE_CURVE ( 'NONE', #756, #9462, #18530, .T. ) ;
#31541=CARTESIAN_POINT ( 'NONE',  ( 64.96297466771235918, -13.74047052604243646, 8.573397087748993783 ) ) ;
#31563=CARTESIAN_POINT ( 'NONE',  ( -14.41812891119675122, -13.74047052604243646, 93.34357519277924098 ) ) ;
#31566=FACE_OUTER_BOUND ( 'NONE', #31374, .T. ) ;
#31573=CARTESIAN_POINT ( 'NONE',  ( 21.09785597605719332, 77.37245976740706510, 47.04930799450051637 ) ) ;
#31588=DIRECTION ( 'NONE',  ( 0.000000000000000000, 1.000000000000000000, -0.000000000000000000 ) ) ;
#31590=EDGE_LOOP ( 'NONE', ( #22760, #29792, #6223, #14554 ) ) ;
#31595=CARTESIAN_POINT ( 'NONE',  ( 21.09785597605720042, -17.03545420775220265, 47.04930799450051637 ) ) ;
#31611=AXIS2_PLACEMENT_3D ( 'NONE', #15064, #2428, #22272 ) ;
#31613=VERTEX_POINT ( 'NONE', #1172 ) ;
#31621=EDGE_CURVE ( 'NONE', #14823, #32191, #25369, .T. ) ;
#31682=EDGE_CURVE ( 'NONE', #14178, #11078, #712, .T. ) ;
#31686=ORIENTED_EDGE ( 'NONE', *, *, #10285, .F. ) ;
#31687=AXIS2_PLACEMENT_3D ( 'NONE', #14314, #11849, #24313 ) ;
#31698=CARTESIAN_POINT ( 'NONE',  ( 71.62639656063521443, -13.74047052604243824, 76.22825493111783146 ) ) ;
#31700=CARTESIAN_POINT ( 'NONE',  ( 21.09785597605719332, 17.16451738380053627, 34.56516646732340092 ) ) ;
#31708=ORIENTED_EDGE ( 'NONE', *, *, #31682, .F. ) ;
#31710=EDGE_CURVE ( 'NONE', #11885, #14867, #24889, .T. ) ;
#31722=CARTESIAN_POINT ( 'NONE',  ( 21.09785597605719332, -13.74048473023143835, 105.2732083928529221 ) ) ;
#31725=DIRECTION ( 'NONE',  ( 0.000000000000000000, 0.000000000000000000, -1.000000000000000000 ) ) ;
#31773=CARTESIAN_POINT ( 'NONE',  ( 21.09785597605721108, -52.14605111273580462, 125.5493079945005093 ) ) ;
#31780=PRODUCT_DEFINITION ( 'UNKNOWN', '', #26538, #18646 ) ;
#31790=EDGE_CURVE ( 'NONE', #8764, #29601, #17551, .T. ) ;
#31793=DIRECTION ( 'NONE',  ( 0.000000000000000000, 0.000000000000000000, -1.000000000000000000 ) ) ;
#31807=DIRECTION ( 'NONE',  ( 0.000000000000000000, -0.000000000000000000, 1.000000000000000000 ) ) ;
#31850=CARTESIAN_POINT ( 'NONE',  ( 28.40365102626034144, -13.30632128221580857, -8.403770473392276230 ) ) ;
#31868=DIRECTION ( 'NONE',  ( 0.000000000000000000, 1.000000000000000000, -0.000000000000000000 ) ) ;
#31879=CARTESIAN_POINT ( 'NONE',  ( -31.23570478744295187, -13.74047052604243646, 21.24731629327110127 ) ) ;
#31897=ORIENTED_EDGE ( 'NONE', *, *, #14617, .T. ) ;
#31935=EDGE_CURVE ( 'NONE', #12577, #756, #22249, .T. ) ;
#31940=ADVANCED_FACE ( 'NONE', ( #27856 ), #23821, .F. ) ;
#31950=CIRCLE ( 'NONE', #16757, 13.23540278830031447 ) ;
#31951=CIRCLE ( 'NONE', #26188, 94.94530576803616384 ) ;
#31963=DIRECTION ( 'NONE',  ( -1.000000000000000000, 0.000000000000000000, 0.000000000000000000 ) ) ;
#31986=ORIENTED_EDGE ( 'NONE', *, *, #9031, .T. ) ;
#32007=DIRECTION ( 'NONE',  ( 1.000000000000000000, 0.000000000000000000, 0.000000000000000000 ) ) ;
#32015=TOROIDAL_SURFACE ( 'NONE', #17861, 13.98419020052803852, 1.000000000001014744 ) ;
#32018=CARTESIAN_POINT ( 'NONE',  ( 21.09785597605720753, -13.56320000832927875, -8.579118024061138215 ) ) ;
#32020=CARTESIAN_POINT ( 'NONE',  ( 59.57376688280871235, -13.74047052604243468, 90.91442668615565026 ) ) ;
#32021=ORIENTED_EDGE ( 'NONE', *, *, #26529, .F. ) ;
#32022=DIRECTION ( 'NONE',  ( 0.000000000000000000, 0.000000000000000000, -1.000000000000000000 ) ) ;
#32023=AXIS2_PLACEMENT_3D ( 'NONE', #32290, #19796, #29828 ) ;
#32040=DIRECTION ( 'NONE',  ( 0.000000000000000000, 0.000000000000000000, -1.000000000000000000 ) ) ;
#32042=CLOSED_SHELL ( 'NONE', ( #32356, #9817, #24560, #21105, #16620, #9942, #29857, #23124, #27469, #10240, #5560, #27712, #25397, #29729, #15351, #3800, #17377, #8594, #31224, #23167, #27679, #11683, #31940, #30513, #549, #27497, #24480, #6974, #10245, #8931, #19022, #5834, #25447, #7866, #24991, #8572, #10052, #4264, #4607, #8137, #22153, #32471, #9398, #21957, #16553, #4857, #6996, #21471, #9222, #13190, #30628, #17330, #16998, #1806, #1376, #16150, #32442, #6736, #12006, #26294, #18450, #27996, #14638, #15931, #25530, #18802, #15411, #9583, #27547, #26822, #30992, #27084, #29328 ) ) ;
#32047=CARTESIAN_POINT ( 'NONE',  ( -8.081090960560114667, -13.74047052604243646, -3.479232590077480758 ) ) ;
#32053=EDGE_CURVE ( 'NONE', #3864, #756, #31176, .T. ) ;
#32128=ORIENTED_EDGE ( 'NONE', *, *, #15400, .T. ) ;
#32131=CARTESIAN_POINT ( 'NONE',  ( 21.09785597605720042, -16.03545420775220265, 47.04930799450051637 ) ) ;
#32135=CARTESIAN_POINT ( 'NONE',  ( 21.09785597605720042, -16.73545420775220194, -31.35069200549948221 ) ) ;
#32155=AXIS2_PLACEMENT_3D ( 'NONE', #17015, #30169, #27041 ) ;
#32156=AXIS2_PLACEMENT_3D ( 'NONE', #11292, #24074, #21283 ) ;
#32174=DIRECTION ( 'NONE',  ( -0.000000000000000000, -1.000000000000000000, -0.000000000000000000 ) ) ;
#32182=EDGE_LOOP ( 'NONE', ( #22432, #9312, #13108, #29040, #5491 ) ) ;
#32187=DIRECTION ( 'NONE',  ( -0.000000000000000000, -1.000000000000000000, -0.000000000000000000 ) ) ;
#32190=CARTESIAN_POINT ( 'NONE',  ( 28.71925248772582151, -13.74047052604244179, 104.8978920147615383 ) ) ;
#32191=VERTEX_POINT ( 'NONE', #26512 ) ;
#32211=EDGE_CURVE ( 'NONE', #1157, #8655, #3420, .T. ) ;
#32238=DIRECTION ( 'NONE',  ( -0.000000000000000000, -1.000000000000000000, -0.000000000000000000 ) ) ;
#32246=ORIENTED_EDGE ( 'NONE', *, *, #5846, .T. ) ;
#32251=TOROIDAL_SURFACE ( 'NONE', #11817, 55.72393233686778302, 0.09999999999999760469 ) ;
#32268=DIRECTION ( 'NONE',  ( 0.000000000000000000, 0.000000000000000000, -1.000000000000000000 ) ) ;
#32271=FACE_OUTER_BOUND ( 'NONE', #16946, .T. ) ;
#32273=ORIENTED_EDGE ( 'NONE', *, *, #18477, .T. ) ;
#32290=CARTESIAN_POINT ( 'NONE',  ( 21.09785597605720042, -16.03545420775220265, 47.04930799450051637 ) ) ;
#32310=ORIENTED_EDGE ( 'NONE', *, *, #8639, .F. ) ;
#32335=DIRECTION ( 'NONE',  ( -0.000000000000000000, -1.000000000000000000, -0.000000000000000000 ) ) ;
#32353=EDGE_LOOP ( 'NONE', ( #2474, #18283, #3421, #3785 ) ) ;
#32354=FACE_OUTER_BOUND ( 'NONE', #28740, .T. ) ;
#32356=ADVANCED_FACE ( 'NONE', ( #16814 ), #32251, .T. ) ;
#32366=VECTOR ( 'NONE', #1520, 1000.000000000000227 ) ;
#32370=DIRECTION ( 'NONE',  ( 0.000000000000000000, 1.000000000000000000, -0.000000000000000000 ) ) ;
#32376=SURFACE_SIDE_STYLE ('',( #22999 ) ) ;
#32388=ORIENTED_EDGE ( 'NONE', *, *, #32053, .F. ) ;
#32402=EDGE_CURVE ( 'NONE', #10039, #6352, #17028, .T. ) ;
#32416=VECTOR ( 'NONE', #6029, 1000.000000000000114 ) ;
#32420=FACE_OUTER_BOUND ( 'NONE', #1163, .T. ) ;
#32423=FACE_OUTER_BOUND ( 'NONE', #5986, .T. ) ;
#32433=DIRECTION ( 'NONE',  ( 0.000000000000000000, 0.000000000000000000, 1.000000000000000000 ) ) ;
#32442=ADVANCED_FACE ( 'NONE', ( #10588 ), #25977, .F. ) ;
#32450=CARTESIAN_POINT ( 'NONE',  ( 21.09785597605719332, -12.82881809906321458, 47.04930799450051637 ) ) ;
#32453=ORIENTED_EDGE ( 'NONE', *, *, #30185, .F. ) ;
#32471=ADVANCED_FACE ( 'NONE', ( #18112, #389 ), #25349, .F. ) ;
#32476=ORIENTED_EDGE ( 'NONE', *, *, #15450, .T. ) ;
#32477=ORIENTED_EDGE ( 'NONE', *, *, #5846, .F. ) ;
#32482=AXIS2_PLACEMENT_3D ( 'NONE', #28312, #5832, #12906 ) ;
#32483=VERTEX_POINT ( 'NONE', #27491 ) ;
#32488=CARTESIAN_POINT ( 'NONE',  ( 21.09785597605719332, -13.74048473023143835, 105.2732083928529221 ) ) ;
#32491=CARTESIAN_POINT ( 'NONE',  ( 21.09785597605719687, 2.299431449832689545, 47.04930799450051637 ) ) ;
#32516=COLOUR_RGB('Light Blue',0.38,0.62,0.78);
#32517=FILL_AREA_STYLE_COLOUR('',#32516);
#32518=FILL_AREA_STYLE('',(#32517));
#32519=SURFACE_STYLE_FILL_AREA(#32518);
#32520=SURFACE_SIDE_STYLE('',(#32519));
#32521=SURFACE_STYLE_USAGE(.BOTH.,#32520);
#32522=PRESENTATION_STYLE_ASSIGNMENT((#32521));
ENDSEC;
END-ISO-10303-21;
